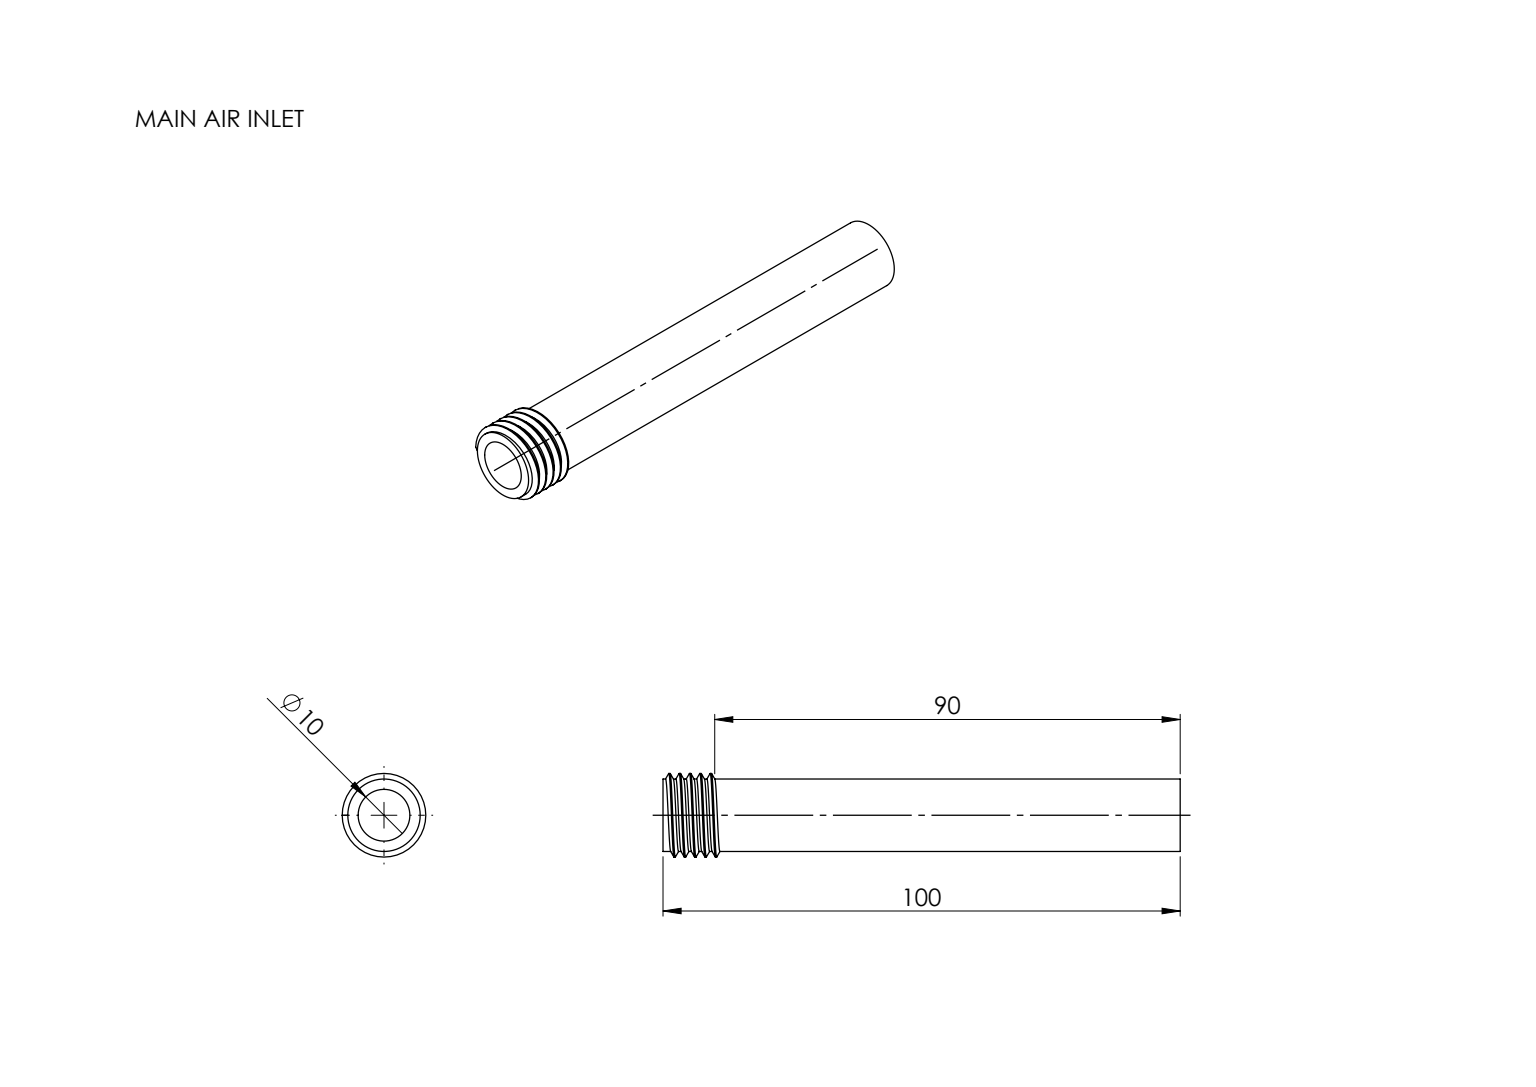
ISO-10303-21;
HEADER;
FILE_DESCRIPTION (('STEP AP214'),
    '1' );
FILE_NAME ('main air inlet.step',
    '2026-10-01T14:18:43',
    ( '' ),
    ( '' ),
    'SwSTEP 2.0',
    'SolidWorks 2026',
    '' );
FILE_SCHEMA (( 'AUTOMOTIVE_DESIGN' ));
ENDSEC;

DATA;
#5=CARTESIAN_POINT ( 'NONE',  ( 95.67376207875069838, 115.9545556584642867, -49.30000000000000426 ) ) ;
#31=CARTESIAN_POINT ( 'NONE',  ( 93.46109445667489979, 105.2492070361643215, -47.42499999726882720 ) ) ;
#33=CARTESIAN_POINT ( 'NONE',  ( 95.00472066334982912, 103.1245878333314323, -47.57499999726882578 ) ) ;
#51=CYLINDRICAL_SURFACE ( 'NONE', #259, 5.000000000000004441 ) ;
#69=CARTESIAN_POINT ( 'NONE',  ( 97.50236033167490746, 102.3130555110000159, -55.22499999726881725 ) ) ;
#81=CARTESIAN_POINT ( 'NONE',  ( 99.99999999999998579, 110.0000000000000000, -145.0000000000000284 ) ) ;
#106=ORIENTED_EDGE ( 'NONE', *, *, #13267, .T. ) ;
#118=EDGE_CURVE ( 'NONE', #27220, #19908, #1908, .T. ) ;
#123=CARTESIAN_POINT ( 'NONE',  ( 92.99999999999998579, 110.0000000000000000, -48.49999999453763877 ) ) ;
#146=CARTESIAN_POINT ( 'NONE',  ( 99.99999999999997158, 102.6397644303321215, -52.50000000000000711 ) ) ;
#174=CARTESIAN_POINT ( 'NONE',  ( 99.99999999999997158, 118.4984768113314146, -52.12499999726881583 ) ) ;
#176=CARTESIAN_POINT ( 'NONE',  ( 106.5389055433250860, 114.7507929638356785, -50.67499999726882010 ) ) ;
#194=CARTESIAN_POINT ( 'NONE',  ( 92.99999999999998579, 110.0000000000000000, -145.0000000000000284 ) ) ;
#209=CARTESIAN_POINT ( 'NONE',  ( 99.99999999999997158, 118.4984768113314004, -52.12499999726880873 ) ) ;
#217=ORIENTED_EDGE ( 'NONE', *, *, #21157, .F. ) ;
#223=CARTESIAN_POINT ( 'NONE',  ( 92.99999999999998579, 110.0000000000000000, -45.00000000000001421 ) ) ;
#257=CARTESIAN_POINT ( 'NONE',  ( 104.9952793366501567, 116.8754121666685393, -48.57499999726882578 ) ) ;
#259=AXIS2_PLACEMENT_3D ( 'NONE', #9021, #6875, #19848 ) ;
#265=CARTESIAN_POINT ( 'NONE',  ( 95.67376207875072680, 104.0454443415356991, -48.19999999453764161 ) ) ;
#289=CARTESIAN_POINT ( 'NONE',  ( 92.99999999999998579, 110.0000000000000000, -53.00000000000001421 ) ) ;
#301=CARTESIAN_POINT ( 'NONE',  ( 92.99999999999998579, 110.0000000000000000, -145.0000000000000284 ) ) ;
#315=CARTESIAN_POINT ( 'NONE',  ( 106.5389055433250860, 105.2492070361643215, -50.82499999726882578 ) ) ;
#317=CARTESIAN_POINT ( 'NONE',  ( 108.0825317499999869, 107.3738262389971538, -54.97499999726881015 ) ) ;
#353=CARTESIAN_POINT ( 'NONE',  ( 93.46109445667489979, 105.2492070361643215, -55.42499999726882720 ) ) ;
#376=ORIENTED_EDGE ( 'NONE', *, *, #19099, .T. ) ;
#388=LINE ( 'NONE', #2390, #9039 ) ;
#389=CARTESIAN_POINT ( 'NONE',  ( 95.67376207875072680, 115.9545556584642867, -54.79999999453764303 ) ) ;
#393=CARTESIAN_POINT ( 'NONE',  ( 106.9999999999999858, 112.2744378736303474, -51.90000000000001279 ) ) ;
#403=CARTESIAN_POINT ( 'NONE',  ( 102.4976396683250783, 117.6869444889999841, -46.47499999726882436 ) ) ;
#431=CARTESIAN_POINT ( 'NONE',  ( 95.67376207875069838, 115.9545556584642867, -47.30000000000000426 ) ) ;
#458=CARTESIAN_POINT ( 'NONE',  ( 97.50236033167490746, 117.6869444889999841, -50.02499999726882152 ) ) ;
#461=CARTESIAN_POINT ( 'NONE',  ( 92.99999999999998579, 110.0000000000000000, -48.49999999453763877 ) ) ;
#498=CARTESIAN_POINT ( 'NONE',  ( 91.91746824999998466, 110.0000000000000000, -53.62499999726882294 ) ) ;
#499=VERTEX_POINT ( 'NONE', #223 ) ;
#530=CARTESIAN_POINT ( 'NONE',  ( 107.0000000000000000, 110.0000000000000000, -55.49999999453763877 ) ) ;
#576=CARTESIAN_POINT ( 'NONE',  ( 95.67376207875069838, 104.0454443415356991, -50.70000000000000284 ) ) ;
#583=ORIENTED_EDGE ( 'NONE', *, *, #5538, .F. ) ;
#600=CARTESIAN_POINT ( 'NONE',  ( 95.00472066334981491, 103.1245878333314465, -51.32499999726881157 ) ) ;
#640=CARTESIAN_POINT ( 'NONE',  ( 102.4976396683250783, 117.6869444889999841, -50.47499999726882436 ) ) ;
#642=VECTOR ( 'NONE', #23365, 1000.000000000000000 ) ;
#674=CARTESIAN_POINT ( 'NONE',  ( 97.83688103937535629, 116.6573956140660897, -52.89999999453764445 ) ) ;
#679=CARTESIAN_POINT ( 'NONE',  ( 104.3262379212492448, 115.9545556584642867, -51.70000000000001705 ) ) ;
#688=CARTESIAN_POINT ( 'NONE',  ( 99.99999999999997158, 101.5015231886685712, -53.37499999726883004 ) ) ;
#699=CARTESIAN_POINT ( 'NONE',  ( 94.33688103937534208, 114.1144967660473242, -45.20000000000000995 ) ) ;
#714=CARTESIAN_POINT ( 'NONE',  ( 97.83688103937535629, 116.6573956140660897, -47.40000000000001279 ) ) ;
#718=CARTESIAN_POINT ( 'NONE',  ( 91.91746824999997045, 112.6261737610028320, -45.72499999726882436 ) ) ;
#722=ORIENTED_EDGE ( 'NONE', *, *, #13713, .T. ) ;
#785=CARTESIAN_POINT ( 'NONE',  ( 97.50236033167490746, 102.3130555110000159, -51.47499999726882436 ) ) ;
#789=VERTEX_POINT ( 'NONE', #17249 ) ;
#836=CARTESIAN_POINT ( 'NONE',  ( 108.0825317499999869, 107.3738262389971680, -54.97499999726881015 ) ) ;
#840=CARTESIAN_POINT ( 'NONE',  ( 99.99999999999997158, 102.6397644303321215, -52.50000000000000711 ) ) ;
#863=CARTESIAN_POINT ( 'NONE',  ( 92.99999999999998579, 110.0000000000000000, -54.49999999453763877 ) ) ;
#868=CARTESIAN_POINT ( 'NONE',  ( 97.50236033167490746, 117.6869444889999841, -50.02499999726882152 ) ) ;
#928=CARTESIAN_POINT ( 'NONE',  ( 93.46109445667489979, 114.7507929638356785, -48.07499999726882578 ) ) ;
#939=DIRECTION ( 'NONE',  ( 1.000000000000000000, 0.000000000000000000, 0.000000000000000000 ) ) ;
#956=EDGE_CURVE ( 'NONE', #3776, #27236, #5144, .T. ) ;
#960=CARTESIAN_POINT ( 'NONE',  ( 92.99999999999998579, 110.0000000000000000, -53.00000000000001421 ) ) ;
#979=CARTESIAN_POINT ( 'NONE',  ( 91.91746824999997045, 112.6261737610028320, -53.97499999726881725 ) ) ;
#1001=CARTESIAN_POINT ( 'NONE',  ( 93.00000000000000000, 112.2744378736303332, -46.59999999453763309 ) ) ;
#1011=CARTESIAN_POINT ( 'NONE',  ( 97.50236033167490746, 117.6869444889999841, -48.02499999726882152 ) ) ;
#1036=CARTESIAN_POINT ( 'NONE',  ( 108.0825317499999869, 112.6261737610028320, -54.52499999726881441 ) ) ;
#1059=DIRECTION ( 'NONE',  ( -1.000000000000000000, 0.000000000000000000, 0.000000000000000000 ) ) ;
#1071=CARTESIAN_POINT ( 'NONE',  ( 106.5389055433250860, 114.7507929638356785, -46.67499999726882720 ) ) ;
#1075=CARTESIAN_POINT ( 'NONE',  ( 107.0000000000000000, 112.2744378736303332, -45.89999999999999858 ) ) ;
#1118=CARTESIAN_POINT ( 'NONE',  ( 91.91746824999997045, 112.6261737610028320, -51.97499999726882436 ) ) ;
#1141=CARTESIAN_POINT ( 'NONE',  ( 107.0000000000000000, 110.0000000000000000, -46.00000000000001421 ) ) ;
#1144=CARTESIAN_POINT ( 'NONE',  ( 102.4976396683250783, 117.6869444889999841, -54.47499999726881725 ) ) ;
#1154=CARTESIAN_POINT ( 'NONE',  ( 104.3262379212492448, 115.9545556584642867, -53.70000000000000284 ) ) ;
#1213=CARTESIAN_POINT ( 'NONE',  ( 108.0825317500000011, 110.0000000000000000, -46.87499999726882294 ) ) ;
#1227=CIRCLE ( 'NONE', #17124, 7.000000000000006217 ) ;
#1256=CARTESIAN_POINT ( 'NONE',  ( 93.46109445667489979, 114.7507929638356785, -52.07499999726881867 ) ) ;
#1274=CARTESIAN_POINT ( 'NONE',  ( 104.3262379212492448, 104.0454443415356991, -46.30000000000001137 ) ) ;
#1277=CARTESIAN_POINT ( 'NONE',  ( 99.99999999999997158, 118.4984768113314004, -54.37499999726880873 ) ) ;
#1285=CARTESIAN_POINT ( 'NONE',  ( 102.4976396683250783, 102.3130555110000159, -47.02499999726882152 ) ) ;
#1289=ORIENTED_EDGE ( 'NONE', *, *, #10160, .T. ) ;
#1354=STYLED_ITEM ( 'NONE', ( #12417 ), #7649 ) ;
#1380=CARTESIAN_POINT ( 'NONE',  ( 97.50236033167490746, 117.6869444889999841, -46.02499999726882152 ) ) ;
#1418=CARTESIAN_POINT ( 'NONE',  ( 92.99999999999998579, 110.0000000000000000, -52.49999999453763877 ) ) ;
#1428=VERTEX_POINT ( 'NONE', #14617 ) ;
#1458=ORIENTED_EDGE ( 'NONE', *, *, #9332, .T. ) ;
#1473=CARTESIAN_POINT ( 'NONE',  ( 93.00000000000001421, 107.7255621263696241, -50.90000000000001279 ) ) ;
#1487=CARTESIAN_POINT ( 'NONE',  ( 102.4976396683250783, 102.3130555110000159, -53.27499999726882862 ) ) ;
#1492=EDGE_CURVE ( 'NONE', #8895, #21015, #19189, .T. ) ;
#1548=CARTESIAN_POINT ( 'NONE',  ( 104.3262379212492448, 104.0454443415356991, -49.79999999453762882 ) ) ;
#1559=CARTESIAN_POINT ( 'NONE',  ( 107.0000000000000000, 107.7255621263696668, -49.59999999453764019 ) ) ;
#1563=CARTESIAN_POINT ( 'NONE',  ( 93.00000000000001421, 107.7255621263696241, -52.39999999453765156 ) ) ;
#1568=CARTESIAN_POINT ( 'NONE',  ( 106.5389055433250860, 105.2492070361643215, -54.82499999726882578 ) ) ;
#1575=CARTESIAN_POINT ( 'NONE',  ( 92.99999999999998579, 110.0000000000000000, -145.0000000000000284 ) ) ;
#1600=ADVANCED_FACE ( 'NONE', ( #7157 ), #15853, .T. ) ;
#1651=CARTESIAN_POINT ( 'NONE',  ( 106.5389055433250860, 114.7507929638356785, -46.42499999726882720 ) ) ;
#1652=EDGE_LOOP ( 'NONE', ( #21390, #1458 ) ) ;
#1665=VECTOR ( 'NONE', #12127, 1000.000000000000000 ) ;
#1675=EDGE_CURVE ( 'NONE', #8859, #12248, #1227, .T. ) ;
#1689=DIRECTION ( 'NONE',  ( 5.782411586589358625E-17, -0.000000000000000000, 1.000000000000000000 ) ) ;
#1691=CIRCLE ( 'NONE', #24441, 7.000000000000006217 ) ;
#1694=CARTESIAN_POINT ( 'NONE',  ( 107.0000000000000000, 110.0000000000000000, -53.49999999453763877 ) ) ;
#1702=CARTESIAN_POINT ( 'NONE',  ( 106.5389055433250860, 114.7507929638356785, -50.42499999726882010 ) ) ;
#1710=EDGE_CURVE ( 'NONE', #11248, #1428, #16566, .T. ) ;
#1732=CARTESIAN_POINT ( 'NONE',  ( 107.0000000000000000, 107.7255621263696668, -46.10000000000000142 ) ) ;
#1749=DIRECTION ( 'NONE',  ( -0.000000000000000000, -0.000000000000000000, -1.000000000000000000 ) ) ;
#1764=CARTESIAN_POINT ( 'NONE',  ( 93.46109445667489979, 105.2492070361643215, -55.67499999726882720 ) ) ;
#1772=ORIENTED_EDGE ( 'NONE', *, *, #956, .T. ) ;
#1779=CARTESIAN_POINT ( 'NONE',  ( 104.3262379212492448, 115.9545556584642867, -47.19999999453763451 ) ) ;
#1829=EDGE_CURVE ( 'NONE', #20267, #3776, #7205, .T. ) ;
#1832=CARTESIAN_POINT ( 'NONE',  ( 95.67376207875069838, 115.9545556584642867, -54.79999999453764303 ) ) ;
#1842=CARTESIAN_POINT ( 'NONE',  ( 104.9952793366501709, 103.1245878333314323, -54.92499999726882720 ) ) ;
#1849=CARTESIAN_POINT ( 'NONE',  ( 107.0000000000000000, 110.0000000000000000, -52.00000000000001421 ) ) ;
#1873=CARTESIAN_POINT ( 'NONE',  ( 97.83688103937537051, 103.3426043859339103, -46.60000000000000853 ) ) ;
#1900=CARTESIAN_POINT ( 'NONE',  ( 91.91746824999997045, 107.3738262389971538, -47.77499999726880731 ) ) ;
#1908=( BOUNDED_CURVE ( )  B_SPLINE_CURVE ( 2, ( #9226, #22347, #21928, #19919, #17490, #13339, #403, #26188, #17781, #11486, #9086, #2404, #6798, #6519, #20202, #15340, #26629, #26484, #6654, #24055, #8661, #15484, #19774, #6939, #4677, #26049, #22066, #257, #4965, #8941, #7077, #15194, #10925, #23912, #13482, #4393, #21785, #17630, #2265, #15635, #2544, #11205, #24335, #4822, #7506, #18057, #9505, #26772, #12046, #9363, #7654, #5529, #24624, #27336, #14195, #7216, #20635, #22914, #11912, #12184, #18495, #1118, #1256, #25179, #5667, #3376, #20771, #20351, #9646, #15906, #20496, #3526, #5101, #18206, #18633, #688, #2954, #9917, #23051, #14056, #7796, #979, #13908, #7360, #16483, #14331, #5243, #9786, #26915, #5386, #27202, #836, #16346, #13765, #25045, #22636, #27056, #22488, #11627, #16053, #24763 ),
 .UNSPECIFIED., .F., .T. ) 
 B_SPLINE_CURVE_WITH_KNOTS ( ( 3, 2, 2, 2, 2, 2, 2, 2, 2, 2, 2, 2, 2, 2, 2, 2, 2, 2, 2, 2, 2, 2, 2, 2, 2, 2, 2, 2, 2, 2, 2, 2, 2, 2, 2, 2, 2, 2, 2, 2, 2, 2, 2, 2, 2, 2, 2, 2, 2, 2, 3 ),
 ( 0.000000000000000000, 0.02000000000000000042, 0.04000000000000000083, 0.05999999999999999778, 0.08000000000000000167, 0.1000000000000000056, 0.1199999999999999956, 0.1400000000000000133, 0.1600000000000000033, 0.1799999999999999933, 0.2000000000000000111, 0.2200000000000000011, 0.2399999999999999911, 0.2600000000000000089, 0.2800000000000000266, 0.2999999999999999889, 0.3200000000000000067, 0.3400000000000000244, 0.3599999999999999867, 0.3800000000000000044, 0.4000000000000000222, 0.4199999999999999845, 0.4400000000000000022, 0.4600000000000000200, 0.4799999999999999822, 0.5000000000000000000, 0.5200000000000000178, 0.5400000000000000355, 0.5600000000000000533, 0.5799999999999999600, 0.5999999999999999778, 0.6199999999999999956, 0.6400000000000000133, 0.6600000000000000311, 0.6800000000000000488, 0.6999999999999999556, 0.7199999999999999734, 0.7399999999999999911, 0.7600000000000000089, 0.7800000000000000266, 0.8000000000000000444, 0.8199999999999999512, 0.8399999999999999689, 0.8599999999999999867, 0.8800000000000000044, 0.9000000000000000222, 0.9200000000000000400, 0.9399999999999999467, 0.9599999999999999645, 0.9799999999999999822, 1.000000000000000000 ),
 .UNSPECIFIED. ) 
 CURVE ( )  GEOMETRIC_REPRESENTATION_ITEM ( )  RATIONAL_B_SPLINE_CURVE ( ( 1.000000000000000000, 0.9510565162951535312, 1.000000000000000000, 0.9510565162951535312, 1.000000000000000000, 0.9510565162951535312, 1.000000000000000000, 0.9510565162951535312, 1.000000000000000000, 0.9510565162951535312, 1.000000000000000000, 0.9510565162951535312, 1.000000000000000000, 0.9510565162951535312, 1.000000000000000000, 0.9510565162951535312, 1.000000000000000000, 0.9510565162951535312, 1.000000000000000000, 0.9510565162951535312, 1.000000000000000000, 0.9510565162951535312, 1.000000000000000000, 0.9510565162951535312, 1.000000000000000000, 0.9510565162951535312, 1.000000000000000000, 0.9510565162951535312, 1.000000000000000000, 0.9510565162951535312, 1.000000000000000000, 0.9510565162951535312, 1.000000000000000000, 0.9510565162951535312, 1.000000000000000000, 0.9510565162951535312, 1.000000000000000000, 0.9510565162951535312, 1.000000000000000000, 0.9510565162951535312, 1.000000000000000000, 0.9510565162951535312, 1.000000000000000000, 0.9510565162951535312, 1.000000000000000000, 0.9510565162951535312, 1.000000000000000000, 0.9510565162951535312, 1.000000000000000000, 0.9510565162951535312, 1.000000000000000000, 0.9510565162951535312, 1.000000000000000000, 0.9510565162951535312, 1.000000000000000000, 0.9510565162951535312, 1.000000000000000000, 0.9510565162951535312, 1.000000000000000000, 0.9510565162951535312, 1.000000000000000000, 0.9510565162951535312, 1.000000000000000000, 0.9510565162951535312, 1.000000000000000000, 0.9510565162951535312, 1.000000000000000000, 0.9510565162951535312, 1.000000000000000000, 0.9510565162951535312, 1.000000000000000000, 0.9510565162951535312, 1.000000000000000000, 0.9510565162951535312, 1.000000000000000000, 0.9510565162951535312, 1.000000000000000000, 0.9510565162951535312, 1.000000000000000000, 0.9510565162951535312, 1.000000000000000000, 0.9510565162951535312, 1.000000000000000000, 0.9510565162951535312, 1.000000000000000000, 0.9510565162951535312, 1.000000000000000000, 0.9510565162951535312, 1.000000000000000000, 0.9510565162951535312, 1.000000000000000000, 0.9510565162951535312, 1.000000000000000000, 0.9510565162951535312, 1.000000000000000000, 0.9510565162951535312, 1.000000000000000000, 0.9510565162951535312, 1.000000000000000000, 0.9510565162951535312, 1.000000000000000000 ) ) 
 REPRESENTATION_ITEM ( '' )  );
#1922=VERTEX_POINT ( 'NONE', #16975 ) ;
#1932=CARTESIAN_POINT ( 'NONE',  ( 91.91746824999997045, 112.6261737610028320, -47.72499999726881725 ) ) ;
#1964=FACE_OUTER_BOUND ( 'NONE', #11666, .T. ) ;
#1966=CARTESIAN_POINT ( 'NONE',  ( 97.83688103937537051, 103.3426043859339103, -54.09999999453764019 ) ) ;
#1969=CARTESIAN_POINT ( 'NONE',  ( 92.99999999999998579, 107.7255621263696526, -56.39999999453763024 ) ) ;
#1974=CARTESIAN_POINT ( 'NONE',  ( 102.4976396683250783, 117.6869444889999841, -50.22499999726882436 ) ) ;
#2032=ADVANCED_FACE ( 'NONE', ( #10693 ), #23546, .T. ) ;
#2033=CARTESIAN_POINT ( 'NONE',  ( 97.50236033167490746, 117.6869444889999841, -46.27499999726882152 ) ) ;
#2043=CARTESIAN_POINT ( 'NONE',  ( 92.99999999999998579, 107.7255621263696526, -54.90000000000001279 ) ) ;
#2067=CARTESIAN_POINT ( 'NONE',  ( 104.9952793366501709, 103.1245878333314323, -52.92499999726882010 ) ) ;
#2103=CARTESIAN_POINT ( 'NONE',  ( 92.99999999999998579, 110.0000000000000000, -56.49999999453763877 ) ) ;
#2118=DIRECTION ( 'NONE',  ( 5.782411586589358625E-17, -0.000000000000000000, 1.000000000000000000 ) ) ;
#2123=CARTESIAN_POINT ( 'NONE',  ( 94.33688103937535629, 105.8855032339526758, -48.29999999453764303 ) ) ;
#2147=CARTESIAN_POINT ( 'NONE',  ( 107.0000000000000000, 112.2744378736303332, -47.90000000000000568 ) ) ;
#2173=CARTESIAN_POINT ( 'NONE',  ( 104.9952793366501567, 103.1245878333314465, -48.92499999726882010 ) ) ;
#2175=CARTESIAN_POINT ( 'NONE',  ( 93.46109445667489979, 105.2492070361643215, -47.67499999726882720 ) ) ;
#2197=CARTESIAN_POINT ( 'NONE',  ( 99.99999999999998579, 110.0000000000000000, -145.0000000000000284 ) ) ;
#2201=ORIENTED_EDGE ( 'NONE', *, *, #6469, .F. ) ;
#2212=CARTESIAN_POINT ( 'NONE',  ( 102.4976396683250783, 102.3130555110000159, -55.02499999726882152 ) ) ;
#2265=CARTESIAN_POINT ( 'NONE',  ( 93.46109445667489979, 105.2492070361643215, -49.67499999726882010 ) ) ;
#2293=CARTESIAN_POINT ( 'NONE',  ( 107.0000000000000000, 107.7255621263696668, -52.10000000000001563 ) ) ;
#2318=CARTESIAN_POINT ( 'NONE',  ( 91.91746824999997045, 112.6261737610028320, -51.72499999726882436 ) ) ;
#2320=CARTESIAN_POINT ( 'NONE',  ( 91.91746824999998466, 110.0000000000000000, -47.87499999726882294 ) ) ;
#2355=CARTESIAN_POINT ( 'NONE',  ( 106.5389055433250860, 114.7507929638356785, -54.42499999726882720 ) ) ;
#2371=( BOUNDED_CURVE ( )  B_SPLINE_CURVE ( 2, ( #25636, #23648, #27790, #14928, #4123, #8248, #21506, #27653, #12788, #6119, #19361 ),
 .UNSPECIFIED., .F., .F. ) 
 B_SPLINE_CURVE_WITH_KNOTS ( ( 3, 2, 2, 2, 2, 3 ),
 ( 0.3000000000000002109, 0.3200000000000002287, 0.3400000000000003020, 0.3600000000000002642, 0.3800000000000003375, 0.4000000000000003553 ),
 .UNSPECIFIED. ) 
 CURVE ( )  GEOMETRIC_REPRESENTATION_ITEM ( )  RATIONAL_B_SPLINE_CURVE ( ( 0.9999999999999994449, 0.9510565162951540863, 1.000000000000000000, 0.9510565162951535312, 1.000000000000000000, 0.9510565162951535312, 1.000000000000000000, 0.9510565162951535312, 1.000000000000000000, 0.9510565162951527540, 1.000000000000000888 ) ) 
 REPRESENTATION_ITEM ( '' )  );
#2390=CARTESIAN_POINT ( 'NONE',  ( 107.0000000000000000, 110.0000000000000000, -145.0000000000000284 ) ) ;
#2394=ORIENTED_EDGE ( 'NONE', *, *, #2626, .F. ) ;
#2404=CARTESIAN_POINT ( 'NONE',  ( 108.0825317499999869, 107.3738262389971680, -46.97499999726881015 ) ) ;
#2433=CARTESIAN_POINT ( 'NONE',  ( 94.33688103937534208, 114.1144967660473242, -47.20000000000000995 ) ) ;
#2454=CARTESIAN_POINT ( 'NONE',  ( 97.50236033167490746, 102.3130555110000159, -49.22499999726882436 ) ) ;
#2456=CARTESIAN_POINT ( 'NONE',  ( 97.50236033167490746, 117.6869444889999841, -48.27499999726882152 ) ) ;
#2490=CARTESIAN_POINT ( 'NONE',  ( 91.91746824999997045, 112.6261737610028320, -51.72499999726882436 ) ) ;
#2544=CARTESIAN_POINT ( 'NONE',  ( 91.91746824999998466, 110.0000000000000000, -49.87499999726882294 ) ) ;
#2574=CARTESIAN_POINT ( 'NONE',  ( 99.99999999999997158, 117.3602355696678501, -51.50000000000001421 ) ) ;
#2581=VERTEX_POINT ( 'NONE', #10035 ) ;
#2599=CARTESIAN_POINT ( 'NONE',  ( 104.9952793366501567, 116.8754121666685393, -48.32499999726882578 ) ) ;
#2601=CARTESIAN_POINT ( 'NONE',  ( 95.67376207875069838, 104.0454443415356991, -48.19999999453764161 ) ) ;
#2626=EDGE_CURVE ( 'NONE', #499, #9571, #1691, .T. ) ;
#2635=CARTESIAN_POINT ( 'NONE',  ( 99.99999999999997158, 101.5015231886685854, -55.12499999726880873 ) ) ;
#2717=CARTESIAN_POINT ( 'NONE',  ( 107.0000000000000000, 107.7255621263696668, -50.10000000000001563 ) ) ;
#2738=CARTESIAN_POINT ( 'NONE',  ( 97.50236033167490746, 102.3130555110000159, -47.22499999726881725 ) ) ;
#2775=CARTESIAN_POINT ( 'NONE',  ( 99.99999999999997158, 118.4984768113314004, -50.37499999726881583 ) ) ;
#2822=CARTESIAN_POINT ( 'NONE',  ( 107.0000000000000000, 110.0000000000000000, -52.00000000000001421 ) ) ;
#2848=CARTESIAN_POINT ( 'NONE',  ( 99.99999999999997158, 102.6397644303321215, -54.50000000000000711 ) ) ;
#2909=CARTESIAN_POINT ( 'NONE',  ( 108.0825317499999869, 107.3738262389971538, -50.97499999726881015 ) ) ;
#2926=VERTEX_POINT ( 'NONE', #12931 ) ;
#2954=CARTESIAN_POINT ( 'NONE',  ( 97.50236033167490746, 102.3130555110000159, -53.47499999726882436 ) ) ;
#2971=EDGE_CURVE ( 'NONE', #1428, #24121, #25364, .T. ) ;
#2974=ORIENTED_EDGE ( 'NONE', *, *, #1675, .F. ) ;
#2986=CARTESIAN_POINT ( 'NONE',  ( 95.00472066334982912, 103.1245878333314323, -49.32499999726881157 ) ) ;
#2997=EDGE_LOOP ( 'NONE', ( #217, #7719, #21919, #9314 ) ) ;
#3015=CARTESIAN_POINT ( 'NONE',  ( 108.0825317500000011, 110.0000000000000000, -52.62499999726882294 ) ) ;
#3018=DIRECTION ( 'NONE',  ( -1.000000000000000000, 0.000000000000000000, 0.000000000000000000 ) ) ;
#3026=ORIENTED_EDGE ( 'NONE', *, *, #8370, .T. ) ;
#3054=CARTESIAN_POINT ( 'NONE',  ( 91.91746824999997045, 112.6261737610028320, -47.97499999726881725 ) ) ;
#3055=ADVANCED_FACE ( 'NONE', ( #23175 ), #17026, .F. ) ;
#3067=FACE_OUTER_BOUND ( 'NONE', #7175, .T. ) ;
#3079=ORIENTED_EDGE ( 'NONE', *, *, #10203, .T. ) ;
#3108=CARTESIAN_POINT ( 'NONE',  ( 97.83688103937537051, 103.3426043859339103, -52.60000000000001563 ) ) ;
#3130=CARTESIAN_POINT ( 'NONE',  ( 108.0825317500000011, 110.0000000000000000, -54.87499999726882294 ) ) ;
#3138=CARTESIAN_POINT ( 'NONE',  ( 95.00472066334982912, 103.1245878333314323, -47.32499999726881157 ) ) ;
#3161=CARTESIAN_POINT ( 'NONE',  ( 106.5389055433250860, 105.2492070361643215, -54.82499999726882578 ) ) ;
#3194=CARTESIAN_POINT ( 'NONE',  ( 104.9952793366501709, 116.8754121666685393, -52.57499999726881867 ) ) ;
#3253=CARTESIAN_POINT ( 'NONE',  ( 105.6631189606246153, 114.1144967660473242, -51.29999999453763593 ) ) ;
#3269=CARTESIAN_POINT ( 'NONE',  ( 91.91746824999998466, 110.0000000000000000, -53.87499999726882294 ) ) ;
#3277=CARTESIAN_POINT ( 'NONE',  ( 107.0000000000000000, 110.0000000000000000, -54.00000000000001421 ) ) ;
#3302=CARTESIAN_POINT ( 'NONE',  ( 91.91746824999998466, 110.0000000000000000, -53.62499999726882294 ) ) ;
#3307=AXIS2_PLACEMENT_3D ( 'NONE', #21369, #2118, #28196 ) ;
#3322=CARTESIAN_POINT ( 'NONE',  ( 104.3262379212492448, 104.0454443415356991, -50.30000000000001137 ) ) ;
#3335=CARTESIAN_POINT ( 'NONE',  ( 104.9952793366501709, 116.8754121666685393, -46.57499999726881157 ) ) ;
#3337=VERTEX_POINT ( 'NONE', #15403 ) ;
#3376=CARTESIAN_POINT ( 'NONE',  ( 99.99999999999997158, 118.4984768113314146, -52.37499999726881583 ) ) ;
#3377=ORIENTED_EDGE ( 'NONE', *, *, #20172, .T. ) ;
#3402=CARTESIAN_POINT ( 'NONE',  ( 102.4976396683250783, 102.3130555110000159, -53.27499999726882862 ) ) ;
#3404=EDGE_LOOP ( 'NONE', ( #14988, #8739, #722, #24690 ) ) ;
#3412=CARTESIAN_POINT ( 'NONE',  ( 106.5389055433250860, 114.7507929638356785, -46.42499999726882720 ) ) ;
#3430=DIRECTION ( 'NONE',  ( 5.782411586589358625E-17, -0.000000000000000000, 1.000000000000000000 ) ) ;
#3521=DIRECTION ( 'NONE',  ( 0.000000000000000000, 0.000000000000000000, -1.000000000000000000 ) ) ;
#3526=CARTESIAN_POINT ( 'NONE',  ( 108.0825317499999869, 107.3738262389971680, -52.97499999726881725 ) ) ;
#3550=CARTESIAN_POINT ( 'NONE',  ( 107.0000000000000000, 107.7255621263696668, -47.59999999453764019 ) ) ;
#3552=ORIENTED_EDGE ( 'NONE', *, *, #25847, .T. ) ;
#3558=CARTESIAN_POINT ( 'NONE',  ( 97.50236033167490746, 102.3130555110000159, -55.22499999726881725 ) ) ;
#3634=CARTESIAN_POINT ( 'NONE',  ( 107.0000000000000000, 110.0000000000000000, -47.49999999453763877 ) ) ;
#3649=CARTESIAN_POINT ( 'NONE',  ( 102.4976396683250783, 117.6869444889999841, -46.22499999726882436 ) ) ;
#3657=( BOUNDED_CURVE ( )  B_SPLINE_CURVE ( 2, ( #13324, #22189, #21916, #389, #4380, #21772, #10771, #17905, #9071, #26176, #530 ),
 .UNSPECIFIED., .F., .F. ) 
 B_SPLINE_CURVE_WITH_KNOTS ( ( 3, 2, 2, 2, 2, 3 ),
 ( 0.8000000000000000444, 0.8199999999999999512, 0.8399999999999999689, 0.8599999999999999867, 0.8800000000000000044, 0.9000000000000000222 ),
 .UNSPECIFIED. ) 
 CURVE ( )  GEOMETRIC_REPRESENTATION_ITEM ( )  RATIONAL_B_SPLINE_CURVE ( ( 1.000000000000000000, 0.9510565162951535312, 1.000000000000000000, 0.9510565162951535312, 1.000000000000000000, 0.9510565162951535312, 1.000000000000000000, 0.9510565162951535312, 1.000000000000000000, 0.9510565162951535312, 1.000000000000000000 ) ) 
 REPRESENTATION_ITEM ( '' )  );
#3678=CARTESIAN_POINT ( 'NONE',  ( 94.33688103937535629, 105.8855032339526758, -50.29999999453763593 ) ) ;
#3686=CARTESIAN_POINT ( 'NONE',  ( 95.67376207875072680, 104.0454443415356991, -46.70000000000000284 ) ) ;
#3688=DIRECTION ( 'NONE',  ( 5.782411586589358625E-17, -0.000000000000000000, 1.000000000000000000 ) ) ;
#3689=CARTESIAN_POINT ( 'NONE',  ( 94.33688103937534208, 114.1144967660473242, -52.69999999453764161 ) ) ;
#3699=CARTESIAN_POINT ( 'NONE',  ( 108.0825317499999869, 107.3738262389971538, -54.72499999726881015 ) ) ;
#3707=DIRECTION ( 'NONE',  ( 5.782411586589358625E-17, -0.000000000000000000, 1.000000000000000000 ) ) ;
#3729=EDGE_CURVE ( 'NONE', #23665, #499, #24540, .T. ) ;
#3733=ORIENTED_EDGE ( 'NONE', *, *, #2971, .F. ) ;
#3741=EDGE_LOOP ( 'NONE', ( #13883, #19434, #3079, #22446, #17485 ) ) ;
#3759=CARTESIAN_POINT ( 'NONE',  ( 104.9952793366501709, 103.1245878333314323, -53.17499999726882010 ) ) ;
#3776=VERTEX_POINT ( 'NONE', #6135 ) ;
#3786=CARTESIAN_POINT ( 'NONE',  ( 91.91746824999997045, 112.6261737610028320, -49.72499999726881725 ) ) ;
#3795=CARTESIAN_POINT ( 'NONE',  ( 91.91746824999998466, 110.0000000000000000, -45.74999999726882294 ) ) ;
#3806=VECTOR ( 'NONE', #3707, 1000.000000000000000 ) ;
#3822=CARTESIAN_POINT ( 'NONE',  ( 107.0000000000000000, 112.2744378736303332, -49.39999999453763735 ) ) ;
#3830=CARTESIAN_POINT ( 'NONE',  ( 106.5389055433250860, 105.2492070361643215, -52.82499999726881867 ) ) ;
#3898=CYLINDRICAL_SURFACE ( 'NONE', #24842, 7.000000000000006217 ) ;
#3921=DIRECTION ( 'NONE',  ( -1.000000000000000000, 0.000000000000000000, 0.000000000000000000 ) ) ;
#3928=ADVANCED_FACE ( 'NONE', ( #16156 ), #9046, .T. ) ;
#3953=CARTESIAN_POINT ( 'NONE',  ( 93.00000000000001421, 107.7255621263696241, -50.39999999453763024 ) ) ;
#3963=AXIS2_PLACEMENT_3D ( 'NONE', #20723, #23383, #6408 ) ;
#3966=CARTESIAN_POINT ( 'NONE',  ( 93.00000000000000000, 112.2744378736303332, -50.59999999453763309 ) ) ;
#3974=CARTESIAN_POINT ( 'NONE',  ( 108.0825317500000011, 110.0000000000000000, -52.62499999726882294 ) ) ;
#4004=CARTESIAN_POINT ( 'NONE',  ( 104.3262379212492448, 104.0454443415356991, -46.30000000000001847 ) ) ;
#4007=DIRECTION ( 'NONE',  ( 5.782411586589358625E-17, -0.000000000000000000, 1.000000000000000000 ) ) ;
#4031=CARTESIAN_POINT ( 'NONE',  ( 104.9952793366501709, 103.1245878333314323, -47.17499999726881299 ) ) ;
#4033=( BOUNDED_CURVE ( )  B_SPLINE_CURVE ( 2, ( #1141, #7816, #5407, #1274, #20793, #18512, #14218, #3686, #14494, #27219, #11792 ),
 .UNSPECIFIED., .F., .F. ) 
 B_SPLINE_CURVE_WITH_KNOTS ( ( 3, 2, 2, 2, 2, 3 ),
 ( 0.1000000000000000056, 0.1200000000000000233, 0.1400000000000000688, 0.1600000000000001144, 0.1800000000000001044, 0.2000000000000001776 ),
 .UNSPECIFIED. ) 
 CURVE ( )  GEOMETRIC_REPRESENTATION_ITEM ( )  RATIONAL_B_SPLINE_CURVE ( ( 1.000000000000000000, 0.9510565162951535312, 1.000000000000000000, 0.9510565162951535312, 1.000000000000000000, 0.9510565162951535312, 1.000000000000000000, 0.9510565162951535312, 1.000000000000000000, 0.9510565162951530871, 1.000000000000000444 ) ) 
 REPRESENTATION_ITEM ( '' )  );
#4037=CARTESIAN_POINT ( 'NONE',  ( 106.5389055433250860, 105.2492070361643215, -53.07499999726881867 ) ) ;
#4066=MECHANICAL_DESIGN_GEOMETRIC_PRESENTATION_REPRESENTATION('',(#1354),#14062);
#4095=DIRECTION ( 'NONE',  ( 5.782411586589358625E-17, -0.000000000000000000, 1.000000000000000000 ) ) ;
#4102=CARTESIAN_POINT ( 'NONE',  ( 93.00000000000000000, 107.7255621263696526, -50.39999999453763024 ) ) ;
#4111=CARTESIAN_POINT ( 'NONE',  ( 97.50236033167490746, 102.3130555110000159, -53.22499999726882436 ) ) ;
#4118=ADVANCED_FACE ( 'NONE', ( #23667 ), #25775, .F. ) ;
#4123=CARTESIAN_POINT ( 'NONE',  ( 102.1631189606246295, 103.3426043859339103, -48.40000000000001279 ) ) ;
#4171=CARTESIAN_POINT ( 'NONE',  ( 95.00472066334982912, 116.8754121666685393, -46.17499999726882720 ) ) ;
#4179=CARTESIAN_POINT ( 'NONE',  ( 105.6631189606246295, 105.8855032339526758, -54.20000000000000995 ) ) ;
#4219=DIRECTION ( 'NONE',  ( -1.000000000000000000, 0.000000000000000000, 5.782411586589357392E-17 ) ) ;
#4226=CARTESIAN_POINT ( 'NONE',  ( 92.99999999999998579, 110.0000000000000000, -50.49999999453763877 ) ) ;
#4256=CARTESIAN_POINT ( 'NONE',  ( 102.1631189606246295, 103.3426043859339103, -47.89999999453763735 ) ) ;
#4280=CARTESIAN_POINT ( 'NONE',  ( 97.83688103937535629, 116.6573956140660897, -49.40000000000001279 ) ) ;
#4311=CARTESIAN_POINT ( 'NONE',  ( 102.4976396683250783, 102.3130555110000159, -49.27499999726882152 ) ) ;
#4327=DIRECTION ( 'NONE',  ( 1.000000000000000000, 0.000000000000000000, 0.000000000000000000 ) ) ;
#4333=SURFACE_SIDE_STYLE ('',( #23719 ) ) ;
#4340=VECTOR ( 'NONE', #20910, 1000.000000000000114 ) ;
#4343=CARTESIAN_POINT ( 'NONE',  ( 104.9952793366501709, 103.1245878333314323, -50.92499999726882010 ) ) ;
#4358=( BOUNDED_CURVE ( )  B_SPLINE_CURVE ( 2, ( #27634, #10080, #23217, #27771, #18792, #21355, #12356, #25208, #8093, #1563, #27225 ),
 .UNSPECIFIED., .F., .F. ) 
 B_SPLINE_CURVE_WITH_KNOTS ( ( 3, 2, 2, 2, 2, 3 ),
 ( 0.4999999999999996669, 0.5199999999999996847, 0.5399999999999998135, 0.5599999999999998312, 0.5799999999999998490, 0.5999999999999998668 ),
 .UNSPECIFIED. ) 
 CURVE ( )  GEOMETRIC_REPRESENTATION_ITEM ( )  RATIONAL_B_SPLINE_CURVE ( ( 1.000000000000000888, 0.9510565162951527540, 1.000000000000000000, 0.9510565162951535312, 1.000000000000000000, 0.9510565162951535312, 1.000000000000000000, 0.9510565162951535312, 1.000000000000000000, 0.9510565162951537532, 0.9999999999999997780 ) ) 
 REPRESENTATION_ITEM ( '' )  );
#4380=CARTESIAN_POINT ( 'NONE',  ( 97.83688103937535629, 116.6573956140660897, -54.89999999453763735 ) ) ;
#4393=CARTESIAN_POINT ( 'NONE',  ( 99.99999999999997158, 101.5015231886685712, -49.37499999726882294 ) ) ;
#4424=CARTESIAN_POINT ( 'NONE',  ( 104.3262379212492448, 115.9545556584642867, -51.70000000000001705 ) ) ;
#4449=CARTESIAN_POINT ( 'NONE',  ( 106.5389055433250860, 114.7507929638356785, -48.42499999726882010 ) ) ;
#4451=CARTESIAN_POINT ( 'NONE',  ( 104.9952793366501709, 116.8754121666685393, -48.57499999726881867 ) ) ;
#4486=CARTESIAN_POINT ( 'NONE',  ( 91.91746824999997045, 112.6261737610028320, -53.72499999726881725 ) ) ;
#4519=CARTESIAN_POINT ( 'NONE',  ( 104.3262379212492448, 115.9545556584642867, -49.70000000000001705 ) ) ;
#4539=CARTESIAN_POINT ( 'NONE',  ( 92.99999999999998579, 107.7255621263696952, -48.39999999453764445 ) ) ;
#4560=CARTESIAN_POINT ( 'NONE',  ( 94.33688103937534208, 114.1144967660473242, -49.20000000000001705 ) ) ;
#4576=AXIS2_PLACEMENT_3D ( 'NONE', #14901, #19337, #25611 ) ;
#4586=CARTESIAN_POINT ( 'NONE',  ( 102.4976396683250783, 117.6869444889999841, -52.22499999726882436 ) ) ;
#4588=CARTESIAN_POINT ( 'NONE',  ( 106.5389055433250860, 105.2492070361643215, -47.07499999726882578 ) ) ;
#4590=EDGE_CURVE ( 'NONE', #1922, #27220, #27600, .T. ) ;
#4607=ADVANCED_BREP_SHAPE_REPRESENTATION ( '', ( #7649, #26844 ), #10431 ) ;
#4626=CARTESIAN_POINT ( 'NONE',  ( 95.00472066334982912, 116.8754121666685393, -51.92499999726881299 ) ) ;
#4650=ORIENTED_EDGE ( 'NONE', *, *, #15930, .T. ) ;
#4662=CARTESIAN_POINT ( 'NONE',  ( 102.1631189606246295, 103.3426043859339103, -55.89999999453763735 ) ) ;
#4677=CARTESIAN_POINT ( 'NONE',  ( 97.50236033167490746, 117.6869444889999841, -48.27499999726882152 ) ) ;
#4707=CARTESIAN_POINT ( 'NONE',  ( 102.1631189606246295, 103.3426043859339103, -52.40000000000001279 ) ) ;
#4732=CARTESIAN_POINT ( 'NONE',  ( 93.46109445667489979, 114.7507929638356785, -49.82499999726882578 ) ) ;
#4734=CARTESIAN_POINT ( 'NONE',  ( 102.4976396683250783, 117.6869444889999841, -52.47499999726882436 ) ) ;
#4767=CARTESIAN_POINT ( 'NONE',  ( 97.50236033167490746, 102.3130555110000159, -51.22499999726882436 ) ) ;
#4809=CARTESIAN_POINT ( 'NONE',  ( 105.6631189606246153, 114.1144967660473242, -51.80000000000001137 ) ) ;
#4822=CARTESIAN_POINT ( 'NONE',  ( 95.00472066334981491, 116.8754121666685393, -50.17499999726882010 ) ) ;
#4852=CARTESIAN_POINT ( 'NONE',  ( 107.0000000000000000, 110.0000000000000000, -48.00000000000001421 ) ) ;
#4878=CARTESIAN_POINT ( 'NONE',  ( 106.5389055433250860, 114.7507929638356785, -50.42499999726882010 ) ) ;
#4880=CARTESIAN_POINT ( 'NONE',  ( 95.00472066334982912, 103.1245878333314323, -55.57499999726881157 ) ) ;
#4916=CARTESIAN_POINT ( 'NONE',  ( 106.5389055433250860, 105.2492070361643215, -50.82499999726882578 ) ) ;
#4965=CARTESIAN_POINT ( 'NONE',  ( 106.5389055433250860, 114.7507929638356785, -48.67499999726882010 ) ) ;
#4998=CARTESIAN_POINT ( 'NONE',  ( 93.00000000000000000, 107.7255621263696526, -54.90000000000001279 ) ) ;
#5020=CARTESIAN_POINT ( 'NONE',  ( 102.4976396683250783, 102.3130555110000159, -47.02499999726882152 ) ) ;
#5022=AXIS2_PLACEMENT_3D ( 'NONE', #13815, #3430, #9272 ) ;
#5055=CARTESIAN_POINT ( 'NONE',  ( 102.4976396683250783, 117.6869444889999841, -48.47499999726882436 ) ) ;
#5071=( BOUNDED_CURVE ( )  B_SPLINE_CURVE ( 2, ( #11165, #18133, #9434, #12532, #6147, #14676, #27542, #6012, #12258, #5602, #20848 ),
 .UNSPECIFIED., .F., .F. ) 
 B_SPLINE_CURVE_WITH_KNOTS ( ( 3, 2, 2, 2, 2, 3 ),
 ( 0.8000000000000000444, 0.8199999999999999512, 0.8399999999999999689, 0.8599999999999999867, 0.8800000000000000044, 0.9000000000000000222 ),
 .UNSPECIFIED. ) 
 CURVE ( )  GEOMETRIC_REPRESENTATION_ITEM ( )  RATIONAL_B_SPLINE_CURVE ( ( 1.000000000000000000, 0.9510565162951535312, 1.000000000000000000, 0.9510565162951535312, 1.000000000000000000, 0.9510565162951535312, 1.000000000000000000, 0.9510565162951535312, 1.000000000000000000, 0.9510565162951535312, 1.000000000000000000 ) ) 
 REPRESENTATION_ITEM ( '' )  );
#5101=CARTESIAN_POINT ( 'NONE',  ( 106.5389055433250860, 105.2492070361643215, -53.07499999726881867 ) ) ;
#5131=CARTESIAN_POINT ( 'NONE',  ( 95.00472066334982912, 116.8754121666685393, -47.92499999726882010 ) ) ;
#5144=LINE ( 'NONE', #301, #14401 ) ;
#5153=FACE_OUTER_BOUND ( 'NONE', #3404, .T. ) ;
#5159=CARTESIAN_POINT ( 'NONE',  ( 93.46109445667489979, 114.7507929638356785, -53.82499999726881867 ) ) ;
#5196=CARTESIAN_POINT ( 'NONE',  ( 95.00472066334982912, 116.8754121666685393, -50.17499999726882010 ) ) ;
#5200=ORIENTED_EDGE ( 'NONE', *, *, #16341, .F. ) ;
#5215=ORIENTED_EDGE ( 'NONE', *, *, #1492, .T. ) ;
#5224=CARTESIAN_POINT ( 'NONE',  ( 107.0000000000000000, 110.0000000000000000, -47.49999999453763877 ) ) ;
#5243=CARTESIAN_POINT ( 'NONE',  ( 102.4976396683250783, 117.6869444889999841, -54.47499999726881725 ) ) ;
#5268=CARTESIAN_POINT ( 'NONE',  ( 99.99999999999998579, 110.0000000000000000, -145.0000000000000284 ) ) ;
#5270=CARTESIAN_POINT ( 'NONE',  ( 105.6631189606246153, 114.1144967660473242, -47.80000000000001137 ) ) ;
#5274=CARTESIAN_POINT ( 'NONE',  ( 102.4976396683250783, 117.6869444889999841, -46.22499999726882436 ) ) ;
#5302=CARTESIAN_POINT ( 'NONE',  ( 102.4976396683250783, 102.3130555110000159, -53.02499999726882862 ) ) ;
#5339=CARTESIAN_POINT ( 'NONE',  ( 108.0825317499999869, 107.3738262389971538, -46.97499999726881015 ) ) ;
#5358=ORIENTED_EDGE ( 'NONE', *, *, #16341, .T. ) ;
#5386=CARTESIAN_POINT ( 'NONE',  ( 108.0825317499999869, 112.6261737610028320, -54.77499999726881441 ) ) ;
#5396=DIRECTION ( 'NONE',  ( 5.782411586589358625E-17, -0.000000000000000000, 1.000000000000000000 ) ) ;
#5407=CARTESIAN_POINT ( 'NONE',  ( 105.6631189606246295, 105.8855032339526758, -46.20000000000000995 ) ) ;
#5412=CARTESIAN_POINT ( 'NONE',  ( 93.46109445667489979, 105.2492070361643215, -53.67499999726882720 ) ) ;
#5421=CARTESIAN_POINT ( 'NONE',  ( 97.50236033167490746, 102.3130555110000159, -47.22499999726881725 ) ) ;
#5444=AXIS2_PLACEMENT_3D ( 'NONE', #8711, #21840, #21976 ) ;
#5458=STYLED_ITEM ( 'NONE', ( #10864 ), #4607 ) ;
#5478=CARTESIAN_POINT ( 'NONE',  ( 106.5389055433250860, 114.7507929638356785, -48.67499999726882010 ) ) ;
#5495=EDGE_CURVE ( 'NONE', #27220, #23665, #9503, .T. ) ;
#5501=ORIENTED_EDGE ( 'NONE', *, *, #12587, .T. ) ;
#5512=CARTESIAN_POINT ( 'NONE',  ( 106.9999999999999858, 112.2744378736303474, -53.39999999453764445 ) ) ;
#5529=CARTESIAN_POINT ( 'NONE',  ( 108.0825317499999869, 107.3738262389971680, -50.97499999726881725 ) ) ;
#5536=CARTESIAN_POINT ( 'NONE',  ( 94.33688103937534208, 114.1144967660473242, -50.69999999453764161 ) ) ;
#5538=EDGE_CURVE ( 'NONE', #2926, #21015, #20880, .T. ) ;
#5556=CARTESIAN_POINT ( 'NONE',  ( 106.5389055433250860, 105.2492070361643215, -55.07499999726882578 ) ) ;
#5565=CARTESIAN_POINT ( 'NONE',  ( 99.99999999999997158, 118.4984768113314004, -46.12499999726880873 ) ) ;
#5568=ORIENTED_EDGE ( 'NONE', *, *, #14474, .T. ) ;
#5588=CARTESIAN_POINT ( 'NONE',  ( 104.9952793366501567, 103.1245878333314465, -54.92499999726882720 ) ) ;
#5602=CARTESIAN_POINT ( 'NONE',  ( 107.0000000000000000, 112.2744378736303190, -53.90000000000000568 ) ) ;
#5608=CARTESIAN_POINT ( 'NONE',  ( 105.6631189606246295, 105.8855032339526758, -50.20000000000001705 ) ) ;
#5629=AXIS2_PLACEMENT_3D ( 'NONE', #9750, #16014, #939 ) ;
#5667=CARTESIAN_POINT ( 'NONE',  ( 97.50236033167490746, 117.6869444889999841, -52.27499999726882862 ) ) ;
#5674=DIRECTION ( 'NONE',  ( -0.000000000000000000, -0.000000000000000000, 1.000000000000000000 ) ) ;
#5691=CARTESIAN_POINT ( 'NONE',  ( 102.1631189606246295, 103.3426043859339103, -47.89999999453763735 ) ) ;
#5701=CARTESIAN_POINT ( 'NONE',  ( 91.91746824999998466, 110.0000000000000000, -53.62499999726882294 ) ) ;
#5756=SURFACE_STYLE_FILL_AREA ( #8433 ) ;
#5767=ORIENTED_EDGE ( 'NONE', *, *, #1710, .T. ) ;
#5790=CARTESIAN_POINT ( 'NONE',  ( 99.99999999999997158, 101.5015231886685854, -49.12499999726882294 ) ) ;
#5829=CARTESIAN_POINT ( 'NONE',  ( 95.67376207875069838, 115.9545556584642867, -50.79999999453764303 ) ) ;
#5837=CARTESIAN_POINT ( 'NONE',  ( 93.46109445667489979, 105.2492070361643215, -53.42499999726882720 ) ) ;
#5897=SURFACE_SIDE_STYLE ('',( #5756 ) ) ;
#5916=CARTESIAN_POINT ( 'NONE',  ( 95.67376207875072680, 115.9545556584642867, -46.79999999453764303 ) ) ;
#5928=CARTESIAN_POINT ( 'NONE',  ( 91.91746824999997045, 107.3738262389971538, -49.52499999726881441 ) ) ;
#5962=CARTESIAN_POINT ( 'NONE',  ( 97.83688103937537051, 103.3426043859339103, -52.09999999453764019 ) ) ;
#5972=CARTESIAN_POINT ( 'NONE',  ( 95.00472066334982912, 116.8754121666685393, -53.92499999726881299 ) ) ;
#6012=CARTESIAN_POINT ( 'NONE',  ( 104.3262379212492448, 115.9545556584642867, -53.69999999999999574 ) ) ;
#6040=CARTESIAN_POINT ( 'NONE',  ( 97.83688103937537051, 103.3426043859339103, -54.60000000000000853 ) ) ;
#6056=SURFACE_STYLE_USAGE ( .BOTH. , #4333 ) ;
#6064=CARTESIAN_POINT ( 'NONE',  ( 108.0825317499999869, 112.6261737610028320, -46.52499999726882152 ) ) ;
#6071=EDGE_CURVE ( 'NONE', #16704, #17997, #2371, .T. ) ;
#6079=DIRECTION ( 'NONE',  ( -5.782411586589357392E-17, 0.000000000000000000, -1.000000000000000000 ) ) ;
#6095=CYLINDRICAL_SURFACE ( 'NONE', #4576, 7.000000000000006217 ) ;
#6099=CARTESIAN_POINT ( 'NONE',  ( 107.0000000000000000, 110.0000000000000000, -49.49999999453764588 ) ) ;
#6107=CARTESIAN_POINT ( 'NONE',  ( 95.00472066334982912, 103.1245878333314323, -53.32499999726881157 ) ) ;
#6119=CARTESIAN_POINT ( 'NONE',  ( 92.99999999999997158, 107.7255621263696810, -48.90000000000001279 ) ) ;
#6135=CARTESIAN_POINT ( 'NONE',  ( 92.99999999999998579, 110.0000000000000000, -51.00000000000000711 ) ) ;
#6147=CARTESIAN_POINT ( 'NONE',  ( 97.83688103937535629, 116.6573956140660897, -53.40000000000001990 ) ) ;
#6164=CARTESIAN_POINT ( 'NONE',  ( 108.0825317499999869, 112.6261737610028320, -48.77499999726882152 ) ) ;
#6170=CARTESIAN_POINT ( 'NONE',  ( 91.91746824999997045, 107.3738262389971538, -55.77499999726882862 ) ) ;
#6200=CARTESIAN_POINT ( 'NONE',  ( 91.91746824999997045, 107.3738262389971538, -47.52499999726881441 ) ) ;
#6201=EDGE_CURVE ( 'NONE', #499, #21009, #7037, .T. ) ;
#6237=CARTESIAN_POINT ( 'NONE',  ( 99.99999999999997158, 117.3602355696678501, -54.99999999453763166 ) ) ;
#6241=CARTESIAN_POINT ( 'NONE',  ( 107.0000000000000000, 107.7255621263696668, -55.59999999453764019 ) ) ;
#6245=CARTESIAN_POINT ( 'NONE',  ( 91.91746824999997045, 112.6261737610028320, -51.72499999726882436 ) ) ;
#6298=CARTESIAN_POINT ( 'NONE',  ( 102.4976396683250783, 117.6869444889999841, -50.47499999726882436 ) ) ;
#6309=CARTESIAN_POINT ( 'NONE',  ( 92.99999999999998579, 110.0000000000000000, -55.00000000000002132 ) ) ;
#6333=CARTESIAN_POINT ( 'NONE',  ( 104.9952793366501709, 116.8754121666685393, -48.32499999726881867 ) ) ;
#6352=AXIS2_PLACEMENT_3D ( 'NONE', #20558, #16117, #3018 ) ;
#6371=CARTESIAN_POINT ( 'NONE',  ( 102.1631189606246295, 103.3426043859339103, -53.89999999453763735 ) ) ;
#6408=DIRECTION ( 'NONE',  ( -1.000000000000000000, 0.000000000000000000, 0.000000000000000000 ) ) ;
#6413=CARTESIAN_POINT ( 'NONE',  ( 95.67376207875069838, 115.9545556584642867, -51.30000000000000426 ) ) ;
#6433=( BOUNDED_CURVE ( )  B_SPLINE_CURVE ( 2, ( #9368, #9652, #5536, #25052, #22783, #18502, #7935, #18773, #3253, #7366, #7660 ),
 .UNSPECIFIED., .F., .F. ) 
 B_SPLINE_CURVE_WITH_KNOTS ( ( 3, 2, 2, 2, 2, 3 ),
 ( 0.3999999999999996891, 0.4199999999999996514, 0.4399999999999996692, 0.4599999999999996869, 0.4799999999999996492, 0.4999999999999996669 ),
 .UNSPECIFIED. ) 
 CURVE ( )  GEOMETRIC_REPRESENTATION_ITEM ( )  RATIONAL_B_SPLINE_CURVE ( ( 1.000000000000000888, 0.9510565162951527540, 1.000000000000000000, 0.9510565162951535312, 1.000000000000000000, 0.9510565162951535312, 1.000000000000000000, 0.9510565162951535312, 1.000000000000000000, 0.9510565162951543083, 0.9999999999999992228 ) ) 
 REPRESENTATION_ITEM ( '' )  );
#6440=CARTESIAN_POINT ( 'NONE',  ( 102.4976396683250783, 117.6869444889999841, -46.47499999726882436 ) ) ;
#6448=DIRECTION ( 'NONE',  ( 1.000000000000000000, 0.000000000000000000, 0.000000000000000000 ) ) ;
#6469=EDGE_CURVE ( 'NONE', #10849, #27236, #12847, .T. ) ;
#6472=CARTESIAN_POINT ( 'NONE',  ( 97.50236033167490746, 117.6869444889999841, -50.02499999726882152 ) ) ;
#6503=ORIENTED_EDGE ( 'NONE', *, *, #22032, .T. ) ;
#6519=CARTESIAN_POINT ( 'NONE',  ( 104.9952793366501567, 103.1245878333314465, -47.17499999726882010 ) ) ;
#6546=CARTESIAN_POINT ( 'NONE',  ( 93.00000000000000000, 112.2744378736303332, -51.10000000000000142 ) ) ;
#6570=CARTESIAN_POINT ( 'NONE',  ( 108.0825317499999869, 107.3738262389971680, -50.72499999726881725 ) ) ;
#6572=CARTESIAN_POINT ( 'NONE',  ( 91.91746824999997045, 107.3738262389971538, -49.77499999726881441 ) ) ;
#6581=PLANE ( 'NONE',  #10250 ) ;
#6607=CARTESIAN_POINT ( 'NONE',  ( 97.50236033167490746, 117.6869444889999841, -46.27499999726882152 ) ) ;
#6625=FACE_BOUND ( 'NONE', #1652, .T. ) ;
#6636=CARTESIAN_POINT ( 'NONE',  ( 92.99999999999998579, 110.0000000000000000, -145.0000000000000284 ) ) ;
#6654=CARTESIAN_POINT ( 'NONE',  ( 93.46109445667489979, 105.2492070361643215, -47.67499999726882720 ) ) ;
#6672=FACE_OUTER_BOUND ( 'NONE', #20087, .T. ) ;
#6677=ORIENTED_EDGE ( 'NONE', *, *, #5495, .F. ) ;
#6683=CARTESIAN_POINT ( 'NONE',  ( 107.0000000000000000, 110.0000000000000000, -52.00000000000001421 ) ) ;
#6697=EDGE_CURVE ( 'NONE', #499, #1922, #22610, .T. ) ;
#6710=CARTESIAN_POINT ( 'NONE',  ( 91.91746824999997045, 107.3738262389971680, -47.52499999726881441 ) ) ;
#6713=CARTESIAN_POINT ( 'NONE',  ( 99.99999999999997158, 101.5015231886685854, -51.37499999726882294 ) ) ;
#6749=CARTESIAN_POINT ( 'NONE',  ( 93.46109445667489979, 114.7507929638356785, -49.82499999726882578 ) ) ;
#6752=ORIENTED_EDGE ( 'NONE', *, *, #8600, .F. ) ;
#6798=CARTESIAN_POINT ( 'NONE',  ( 106.5389055433250860, 105.2492070361643215, -47.07499999726882578 ) ) ;
#6828=CARTESIAN_POINT ( 'NONE',  ( 97.83688103937535629, 116.6573956140660897, -47.40000000000001279 ) ) ;
#6833=ORIENTED_EDGE ( 'NONE', *, *, #13516, .T. ) ;
#6852=CARTESIAN_POINT ( 'NONE',  ( 91.91746824999998466, 110.0000000000000000, -47.62499999726882294 ) ) ;
#6854=CARTESIAN_POINT ( 'NONE',  ( 108.0825317499999869, 112.6261737610028320, -52.77499999726883573 ) ) ;
#6866=CARTESIAN_POINT ( 'NONE',  ( 94.33688103937534208, 114.1144967660473242, -48.69999999453764161 ) ) ;
#6875=DIRECTION ( 'NONE',  ( 5.782411586589358625E-17, -0.000000000000000000, 1.000000000000000000 ) ) ;
#6893=CARTESIAN_POINT ( 'NONE',  ( 106.5389055433250860, 114.7507929638356785, -50.42499999726882010 ) ) ;
#6924=CARTESIAN_POINT ( 'NONE',  ( 104.3262379212492448, 104.0454443415356991, -55.79999999453763593 ) ) ;
#6927=EDGE_CURVE ( 'NONE', #3337, #11248, #19368, .T. ) ;
#6939=CARTESIAN_POINT ( 'NONE',  ( 95.00472066334981491, 116.8754121666685393, -48.17499999726882010 ) ) ;
#6970=CARTESIAN_POINT ( 'NONE',  ( 94.33688103937535629, 105.8855032339526758, -46.80000000000001847 ) ) ;
#6994=CARTESIAN_POINT ( 'NONE',  ( 108.0825317499999869, 112.6261737610028320, -46.52499999726882152 ) ) ;
#6996=CARTESIAN_POINT ( 'NONE',  ( 95.67376207875069838, 115.9545556584642867, -46.79999999453764303 ) ) ;
#7003=CARTESIAN_POINT ( 'NONE',  ( 99.99999999999997158, 117.3602355696678643, -48.99999999453763877 ) ) ;
#7026=CARTESIAN_POINT ( 'NONE',  ( 91.91746824999998466, 110.0000000000000000, -45.87499999726882294 ) ) ;
#7031=ORIENTED_EDGE ( 'NONE', *, *, #9332, .F. ) ;
#7037=( BOUNDED_CURVE ( )  B_SPLINE_CURVE ( 2, ( #15496, #24489, #699, #22076, #7228, #19929, #15919, #9096, #19785, #13494, #17791 ),
 .UNSPECIFIED., .F., .T. ) 
 B_SPLINE_CURVE_WITH_KNOTS ( ( 3, 2, 2, 2, 2, 3 ),
 ( 0.000000000000000000, 0.02000000000000000042, 0.04000000000000000083, 0.05999999999999999778, 0.08000000000000000167, 0.1000000000000000194 ),
 .UNSPECIFIED. ) 
 CURVE ( )  GEOMETRIC_REPRESENTATION_ITEM ( )  RATIONAL_B_SPLINE_CURVE ( ( 1.000000000000000000, 0.9510565162951535312, 1.000000000000000000, 0.9510565162951535312, 1.000000000000000000, 0.9510565162951535312, 1.000000000000000000, 0.9510565162951535312, 1.000000000000000000, 0.9510565162951535312, 1.000000000000000000 ) ) 
 REPRESENTATION_ITEM ( '' )  );
#7062=CARTESIAN_POINT ( 'NONE',  ( 105.6631189606246153, 114.1144967660473242, -55.29999999453764303 ) ) ;
#7077=CARTESIAN_POINT ( 'NONE',  ( 108.0825317500000011, 110.0000000000000000, -48.87499999726882294 ) ) ;
#7107=CARTESIAN_POINT ( 'NONE',  ( 99.99999999999997158, 101.5015231886685854, -49.12499999726882294 ) ) ;
#7125=DIRECTION ( 'NONE',  ( -0.8660254037844392627, -0.000000000000000000, 0.4999999999999987788 ) ) ;
#7132=CARTESIAN_POINT ( 'NONE',  ( 104.9952793366501567, 116.8754121666685393, -52.32499999726881867 ) ) ;
#7157=FACE_OUTER_BOUND ( 'NONE', #21496, .T. ) ;
#7167=CARTESIAN_POINT ( 'NONE',  ( 99.99999999999997158, 118.4984768113314004, -46.37499999726880873 ) ) ;
#7175=EDGE_LOOP ( 'NONE', ( #11411, #16309, #5568, #10498 ) ) ;
#7205=( BOUNDED_CURVE ( )  B_SPLINE_CURVE ( 2, ( #20992, #27409, #5608, #3322, #9587, #12267, #7444, #14274, #23272, #1473, #7872 ),
 .UNSPECIFIED., .F., .F. ) 
 B_SPLINE_CURVE_WITH_KNOTS ( ( 3, 2, 2, 2, 2, 3 ),
 ( 0.4999999999999996669, 0.5199999999999996847, 0.5399999999999998135, 0.5599999999999998312, 0.5799999999999998490, 0.5999999999999998668 ),
 .UNSPECIFIED. ) 
 CURVE ( )  GEOMETRIC_REPRESENTATION_ITEM ( )  RATIONAL_B_SPLINE_CURVE ( ( 1.000000000000000888, 0.9510565162951527540, 1.000000000000000000, 0.9510565162951535312, 1.000000000000000000, 0.9510565162951535312, 1.000000000000000000, 0.9510565162951535312, 1.000000000000000000, 0.9510565162951537532, 0.9999999999999997780 ) ) 
 REPRESENTATION_ITEM ( '' )  );
#7214=CIRCLE ( 'NONE', #24976, 7.000000000000006217 ) ;
#7216=CARTESIAN_POINT ( 'NONE',  ( 99.99999999999997158, 101.5015231886685712, -51.37499999726882294 ) ) ;
#7228=CARTESIAN_POINT ( 'NONE',  ( 97.83688103937535629, 116.6573956140660897, -45.40000000000001279 ) ) ;
#7252=CARTESIAN_POINT ( 'NONE',  ( 108.0825317500000011, 110.0000000000000000, -46.62499999726882294 ) ) ;
#7279=VECTOR ( 'NONE', #27154, 1000.000000000000000 ) ;
#7287=CARTESIAN_POINT ( 'NONE',  ( 93.00000000000000000, 112.2744378736303332, -48.59999999453764019 ) ) ;
#7315=CARTESIAN_POINT ( 'NONE',  ( 91.91746824999997045, 112.6261737610028320, -51.97499999726882436 ) ) ;
#7323=VERTEX_POINT ( 'NONE', #5224 ) ;
#7344=CARTESIAN_POINT ( 'NONE',  ( 105.6631189606246153, 114.1144967660473242, -53.29999999453764303 ) ) ;
#7360=CARTESIAN_POINT ( 'NONE',  ( 95.00472066334981491, 116.8754121666685393, -54.17499999726882720 ) ) ;
#7366=CARTESIAN_POINT ( 'NONE',  ( 106.9999999999999716, 112.2744378736303759, -51.39999999453765156 ) ) ;
#7392=CARTESIAN_POINT ( 'NONE',  ( 94.33688103937535629, 105.8855032339526758, -54.80000000000001847 ) ) ;
#7444=CARTESIAN_POINT ( 'NONE',  ( 97.83688103937537051, 103.3426043859339103, -50.60000000000001563 ) ) ;
#7456=CARTESIAN_POINT ( 'NONE',  ( 99.99999999999997158, 101.5015231886685854, -51.37499999726882294 ) ) ;
#7488=CARTESIAN_POINT ( 'NONE',  ( 95.67376207875072680, 115.9545556584642867, -52.79999999453764303 ) ) ;
#7493=CARTESIAN_POINT ( 'NONE',  ( 94.33688103937534208, 114.1144967660473242, -51.20000000000000995 ) ) ;
#7506=CARTESIAN_POINT ( 'NONE',  ( 97.50236033167490746, 117.6869444889999841, -50.27499999726882152 ) ) ;
#7530=CARTESIAN_POINT ( 'NONE',  ( 106.5389055433250860, 114.7507929638356785, -54.67499999726882720 ) ) ;
#7539=CARTESIAN_POINT ( 'NONE',  ( 104.9952793366501709, 103.1245878333314323, -48.92499999726882010 ) ) ;
#7607=CARTESIAN_POINT ( 'NONE',  ( 97.50236033167490746, 102.3130555110000159, -47.47499999726881725 ) ) ;
#7649=MANIFOLD_SOLID_BREP ( 'Thread1', #14440 ) ;
#7654=CARTESIAN_POINT ( 'NONE',  ( 108.0825317500000011, 110.0000000000000000, -50.87499999726882294 ) ) ;
#7660=CARTESIAN_POINT ( 'NONE',  ( 107.0000000000000000, 110.0000000000000000, -51.49999999453763877 ) ) ;
#7676=CARTESIAN_POINT ( 'NONE',  ( 102.4976396683250783, 102.3130555110000159, -55.27499999726882152 ) ) ;
#7683=AXIS2_PLACEMENT_3D ( 'NONE', #21070, #3688, #12481 ) ;
#7685=CARTESIAN_POINT ( 'NONE',  ( 99.99999999999997158, 118.4984768113314004, -48.12499999726881583 ) ) ;
#7713=CARTESIAN_POINT ( 'NONE',  ( 106.5389055433250860, 105.2492070361643215, -52.82499999726881867 ) ) ;
#7719=ORIENTED_EDGE ( 'NONE', *, *, #9595, .T. ) ;
#7741=ORIENTED_EDGE ( 'NONE', *, *, #11083, .T. ) ;
#7746=LINE ( 'NONE', #18853, #7279 ) ;
#7747=CARTESIAN_POINT ( 'NONE',  ( 99.99999999999997158, 101.5015231886685854, -49.37499999726882294 ) ) ;
#7777=LINE ( 'NONE', #12310, #19119 ) ;
#7796=CARTESIAN_POINT ( 'NONE',  ( 91.91746824999998466, 110.0000000000000000, -53.87499999726882294 ) ) ;
#7805=DIRECTION ( 'NONE',  ( 5.782411586589358625E-17, -0.000000000000000000, 1.000000000000000000 ) ) ;
#7816=CARTESIAN_POINT ( 'NONE',  ( 107.0000000000000000, 107.7255621263696668, -46.10000000000000142 ) ) ;
#7820=CARTESIAN_POINT ( 'NONE',  ( 97.50236033167490746, 102.3130555110000159, -53.47499999726882436 ) ) ;
#7827=CARTESIAN_POINT ( 'NONE',  ( 91.91746824999997045, 107.3738262389971538, -51.52499999726882152 ) ) ;
#7872=CARTESIAN_POINT ( 'NONE',  ( 92.99999999999998579, 110.0000000000000000, -51.00000000000000711 ) ) ;
#7884=CARTESIAN_POINT ( 'NONE',  ( 95.00472066334982912, 103.1245878333314323, -55.57499999726881157 ) ) ;
#7893=ORIENTED_EDGE ( 'NONE', *, *, #8047, .F. ) ;
#7914=CARTESIAN_POINT ( 'NONE',  ( 104.9952793366501709, 116.8754121666685393, -46.32499999726881867 ) ) ;
#7935=CARTESIAN_POINT ( 'NONE',  ( 102.1631189606246153, 116.6573956140660897, -51.09999999453764019 ) ) ;
#7936=VECTOR ( 'NONE', #24823, 1000.000000000000000 ) ;
#7951=CARTESIAN_POINT ( 'NONE',  ( 97.83688103937537051, 103.3426043859339103, -50.09999999453764019 ) ) ;
#7959=VECTOR ( 'NONE', #3521, 1000.000000000000000 ) ;
#7960=CARTESIAN_POINT ( 'NONE',  ( 95.00472066334982912, 103.1245878333314323, -51.32499999726880446 ) ) ;
#8047=EDGE_CURVE ( 'NONE', #12248, #8859, #9084, .T. ) ;
#8051=CARTESIAN_POINT ( 'NONE',  ( 97.50236033167490746, 102.3130555110000159, -49.22499999726882436 ) ) ;
#8090=CARTESIAN_POINT ( 'NONE',  ( 102.1631189606246153, 116.6573956140660897, -53.09999999453764019 ) ) ;
#8093=CARTESIAN_POINT ( 'NONE',  ( 94.33688103937535629, 105.8855032339526758, -52.29999999453764303 ) ) ;
#8100=CARTESIAN_POINT ( 'NONE',  ( 106.5389055433250860, 114.7507929638356785, -54.42499999726882720 ) ) ;
#8129=ADVANCED_FACE ( 'NONE', ( #26797 ), #11511, .T. ) ;
#8191=FACE_BOUND ( 'NONE', #20868, .T. ) ;
#8215=CARTESIAN_POINT ( 'NONE',  ( 99.99999999999997158, 102.6397644303321215, -49.99999999453764588 ) ) ;
#8226=CARTESIAN_POINT ( 'NONE',  ( 107.0000000000000000, 112.2744378736303332, -51.39999999453764445 ) ) ;
#8245=EDGE_CURVE ( 'NONE', #24786, #789, #4358, .T. ) ;
#8248=CARTESIAN_POINT ( 'NONE',  ( 99.99999999999997158, 102.6397644303321215, -48.50000000000000711 ) ) ;
#8292=CARTESIAN_POINT ( 'NONE',  ( 102.4976396683250783, 102.3130555110000159, -47.27499999726882152 ) ) ;
#8294=( LENGTH_UNIT ( ) NAMED_UNIT ( * ) SI_UNIT ( .MILLI., .METRE. ) );
#8299=CARTESIAN_POINT ( 'NONE',  ( 104.9952793366501709, 116.8754121666685393, -54.57499999726882578 ) ) ;
#8317=ORIENTED_EDGE ( 'NONE', *, *, #8370, .F. ) ;
#8320=FILL_AREA_STYLE ('',( #8741 ) ) ;
#8329=CARTESIAN_POINT ( 'NONE',  ( 93.46109445667489979, 114.7507929638356785, -45.82499999726881867 ) ) ;
#8362=CARTESIAN_POINT ( 'NONE',  ( 107.0000000000000000, 110.0000000000000000, -145.0000000000000284 ) ) ;
#8366=CARTESIAN_POINT ( 'NONE',  ( 94.33688103937535629, 105.8855032339526758, -52.29999999453764303 ) ) ;
#8370=EDGE_CURVE ( 'NONE', #12194, #15376, #16920, .T. ) ;
#8375=CARTESIAN_POINT ( 'NONE',  ( 104.9952793366501709, 116.8754121666685393, -52.32499999726881867 ) ) ;
#8381=( BOUNDED_SURFACE ( )  B_SPLINE_SURFACE ( 1, 2, ( 
 ( #16983, #21700, #17120, #4171, #2033, #10701, #6440, #10566, #27838, #21559, #21421, #15110, #4588, #4031, #8292, #12968, #23830, #33, #2175, #1900, #2320, #13105, #17408, #25824, #2456, #19552, #11118, #4451, #8858, #6164, #14830, #12832, #10837, #19275, #4311, #13248, #27973, #23554, #26107, #6572, #15255, #23973, #8431, #10977, #21844, #19689, #6298, #14975, #176, #23694, #17549, #26253, #8576, #17266, #25967, #6713, #15399, #24112, #21980, #22939, #14221, #24392, #11796, #19832, #18373, #24926, #4734, #20797, #9811, #6854, #18517, #13394, #9142, #15543, #3402, #27078, #7820, #26399, #5412, #25069, #3269, #9670, #12072, #11937, #20659, #1277, #1144, #24252, #7530, #23074, #3130, #317, #5556, #27361, #7676, #20519, #27222, #4880, #13544, #26540, #16368 ),
 ( #22266, #1001, #9942, #6996, #9005, #16226, #22122, #18657, #15690, #16512, #14080, #3550, #22800, #25205, #5691, #14358, #17697, #2601, #11262, #19983, #461, #17835, #18789, #23761, #27768, #12767, #19340, #21071, #10351, #3822, #6099, #1559, #15044, #20934, #23485, #23626, #7951, #14905, #12626, #4102, #21209, #3966, #25344, #5829, #10077, #25901, #27905, #25484, #28044, #8226, #8511, #14766, #23214, #19060, #25755, #14497, #5962, #12482, #8366, #18922, #1418, #14630, #3689, #10496, #27630, #19203, #8090, #12207, #16785, #23349, #1694, #21485, #17194, #10634, #6371, #25616, #1966, #16916, #27496, #16649, #21352, #12353, #10212, #1832, #17051, #6237, #26325, #13036, #7062, #12897, #15470, #15618, #28180, #6924, #4662, #24320, #13177, #24184, #17339, #26036, #2103 ) ),
 .UNSPECIFIED., .F., .F., .F. ) 
 B_SPLINE_SURFACE_WITH_KNOTS ( ( 2, 2 ),
 ( 3, 2, 2, 2, 2, 2, 2, 2, 2, 2, 2, 2, 2, 2, 2, 2, 2, 2, 2, 2, 2, 2, 2, 2, 2, 2, 2, 2, 2, 2, 2, 2, 2, 2, 2, 2, 2, 2, 2, 2, 2, 2, 2, 2, 2, 2, 2, 2, 2, 2, 3 ),
 ( 0.000000000000000000, 1.000000000000000000 ),
 ( 0.000000000000000000, 0.02000000000000000042, 0.04000000000000000083, 0.05999999999999999778, 0.08000000000000000167, 0.1000000000000000056, 0.1199999999999999956, 0.1400000000000000133, 0.1600000000000000033, 0.1799999999999999933, 0.2000000000000000111, 0.2200000000000000011, 0.2399999999999999911, 0.2600000000000000089, 0.2800000000000000266, 0.2999999999999999889, 0.3200000000000000067, 0.3400000000000000244, 0.3599999999999999867, 0.3800000000000000044, 0.4000000000000000222, 0.4199999999999999845, 0.4400000000000000022, 0.4600000000000000200, 0.4799999999999999822, 0.5000000000000000000, 0.5200000000000000178, 0.5400000000000000355, 0.5600000000000000533, 0.5799999999999999600, 0.5999999999999999778, 0.6199999999999999956, 0.6400000000000000133, 0.6600000000000000311, 0.6800000000000000488, 0.6999999999999999556, 0.7199999999999999734, 0.7399999999999999911, 0.7600000000000000089, 0.7800000000000000266, 0.8000000000000000444, 0.8199999999999999512, 0.8399999999999999689, 0.8599999999999999867, 0.8800000000000000044, 0.9000000000000000222, 0.9200000000000000400, 0.9399999999999999467, 0.9599999999999999645, 0.9799999999999999822, 1.000000000000000000 ),
 .UNSPECIFIED. ) 
 GEOMETRIC_REPRESENTATION_ITEM ( )  RATIONAL_B_SPLINE_SURFACE ( (
 ( 1.000000000000000000, 0.9510565162951535312, 1.000000000000000000, 0.9510565162951535312, 1.000000000000000000, 0.9510565162951535312, 1.000000000000000000, 0.9510565162951535312, 1.000000000000000000, 0.9510565162951535312, 1.000000000000000000, 0.9510565162951535312, 1.000000000000000000, 0.9510565162951535312, 1.000000000000000000, 0.9510565162951535312, 1.000000000000000000, 0.9510565162951535312, 1.000000000000000000, 0.9510565162951535312, 1.000000000000000000, 0.9510565162951535312, 1.000000000000000000, 0.9510565162951535312, 1.000000000000000000, 0.9510565162951535312, 1.000000000000000000, 0.9510565162951535312, 1.000000000000000000, 0.9510565162951535312, 1.000000000000000000, 0.9510565162951535312, 1.000000000000000000, 0.9510565162951535312, 1.000000000000000000, 0.9510565162951535312, 1.000000000000000000, 0.9510565162951535312, 1.000000000000000000, 0.9510565162951535312, 1.000000000000000000, 0.9510565162951535312, 1.000000000000000000, 0.9510565162951535312, 1.000000000000000000, 0.9510565162951535312, 1.000000000000000000, 0.9510565162951535312, 1.000000000000000000, 0.9510565162951535312, 1.000000000000000000, 0.9510565162951535312, 1.000000000000000000, 0.9510565162951535312, 1.000000000000000000, 0.9510565162951535312, 1.000000000000000000, 0.9510565162951535312, 1.000000000000000000, 0.9510565162951535312, 1.000000000000000000, 0.9510565162951535312, 1.000000000000000000, 0.9510565162951535312, 1.000000000000000000, 0.9510565162951535312, 1.000000000000000000, 0.9510565162951535312, 1.000000000000000000, 0.9510565162951535312, 1.000000000000000000, 0.9510565162951535312, 1.000000000000000000, 0.9510565162951535312, 1.000000000000000000, 0.9510565162951535312, 1.000000000000000000, 0.9510565162951535312, 1.000000000000000000, 0.9510565162951535312, 1.000000000000000000, 0.9510565162951535312, 1.000000000000000000, 0.9510565162951535312, 1.000000000000000000, 0.9510565162951535312, 1.000000000000000000, 0.9510565162951535312, 1.000000000000000000, 0.9510565162951535312, 1.000000000000000000, 0.9510565162951535312, 1.000000000000000000, 0.9510565162951535312, 1.000000000000000000, 0.9510565162951535312, 1.000000000000000000, 0.9510565162951535312, 1.000000000000000000, 0.9510565162951535312, 1.000000000000000000),
 ( 1.000000000000000000, 0.9510565162951535312, 1.000000000000000000, 0.9510565162951535312, 1.000000000000000000, 0.9510565162951535312, 1.000000000000000000, 0.9510565162951535312, 1.000000000000000000, 0.9510565162951535312, 1.000000000000000000, 0.9510565162951535312, 1.000000000000000000, 0.9510565162951535312, 1.000000000000000000, 0.9510565162951535312, 1.000000000000000000, 0.9510565162951535312, 1.000000000000000000, 0.9510565162951535312, 1.000000000000000000, 0.9510565162951535312, 1.000000000000000000, 0.9510565162951535312, 1.000000000000000000, 0.9510565162951535312, 1.000000000000000000, 0.9510565162951535312, 1.000000000000000000, 0.9510565162951535312, 1.000000000000000000, 0.9510565162951535312, 1.000000000000000000, 0.9510565162951535312, 1.000000000000000000, 0.9510565162951535312, 1.000000000000000000, 0.9510565162951535312, 1.000000000000000000, 0.9510565162951535312, 1.000000000000000000, 0.9510565162951535312, 1.000000000000000000, 0.9510565162951535312, 1.000000000000000000, 0.9510565162951535312, 1.000000000000000000, 0.9510565162951535312, 1.000000000000000000, 0.9510565162951535312, 1.000000000000000000, 0.9510565162951535312, 1.000000000000000000, 0.9510565162951535312, 1.000000000000000000, 0.9510565162951535312, 1.000000000000000000, 0.9510565162951535312, 1.000000000000000000, 0.9510565162951535312, 1.000000000000000000, 0.9510565162951535312, 1.000000000000000000, 0.9510565162951535312, 1.000000000000000000, 0.9510565162951535312, 1.000000000000000000, 0.9510565162951535312, 1.000000000000000000, 0.9510565162951535312, 1.000000000000000000, 0.9510565162951535312, 1.000000000000000000, 0.9510565162951535312, 1.000000000000000000, 0.9510565162951535312, 1.000000000000000000, 0.9510565162951535312, 1.000000000000000000, 0.9510565162951535312, 1.000000000000000000, 0.9510565162951535312, 1.000000000000000000, 0.9510565162951535312, 1.000000000000000000, 0.9510565162951535312, 1.000000000000000000, 0.9510565162951535312, 1.000000000000000000, 0.9510565162951535312, 1.000000000000000000, 0.9510565162951535312, 1.000000000000000000, 0.9510565162951535312, 1.000000000000000000, 0.9510565162951535312, 1.000000000000000000, 0.9510565162951535312, 1.000000000000000000, 0.9510565162951535312, 1.000000000000000000) ) ) 
 REPRESENTATION_ITEM ( '' )  SURFACE ( )  );
#8398=ORIENTED_EDGE ( 'NONE', *, *, #5495, .T. ) ;
#8405=ORIENTED_EDGE ( 'NONE', *, *, #14283, .F. ) ;
#8429=CARTESIAN_POINT ( 'NONE',  ( 95.00472066334981491, 116.8754121666685393, -45.92499999726882720 ) ) ;
#8431=CARTESIAN_POINT ( 'NONE',  ( 93.46109445667489979, 114.7507929638356785, -50.07499999726882578 ) ) ;
#8433=FILL_AREA_STYLE ('',( #25415 ) ) ;
#8437=CARTESIAN_POINT ( 'NONE',  ( 91.91746824999997045, 112.6261737610028320, -53.97499999726881725 ) ) ;
#8460=( NAMED_UNIT ( * ) PLANE_ANGLE_UNIT ( ) SI_UNIT ( $, .RADIAN. ) );
#8472=CARTESIAN_POINT ( 'NONE',  ( 95.00472066334982912, 116.8754121666685393, -47.92499999726882010 ) ) ;
#8511=CARTESIAN_POINT ( 'NONE',  ( 107.0000000000000000, 110.0000000000000000, -51.49999999453763877 ) ) ;
#8547=CARTESIAN_POINT ( 'NONE',  ( 95.67376207875069838, 115.9545556584642867, -45.30000000000000426 ) ) ;
#8551=LINE ( 'NONE', #17383, #21293 ) ;
#8568=DIRECTION ( 'NONE',  ( 1.000000000000000000, 0.000000000000000000, 0.000000000000000000 ) ) ;
#8571=MECHANICAL_DESIGN_GEOMETRIC_PRESENTATION_REPRESENTATION('',(#5458),#14919);
#8574=CARTESIAN_POINT ( 'NONE',  ( 99.99999999999997158, 118.4984768113314146, -46.12499999726881583 ) ) ;
#8576=CARTESIAN_POINT ( 'NONE',  ( 106.5389055433250860, 105.2492070361643215, -51.07499999726882578 ) ) ;
#8591=DIRECTION ( 'NONE',  ( 1.000000000000000000, 0.000000000000000000, 0.000000000000000000 ) ) ;
#8600=EDGE_CURVE ( 'NONE', #3776, #22871, #25662, .T. ) ;
#8612=CARTESIAN_POINT ( 'NONE',  ( 102.4976396683250783, 117.6869444889999841, -54.22499999726881725 ) ) ;
#8635=CARTESIAN_POINT ( 'NONE',  ( 0.000000000000000000, 0.000000000000000000, 0.000000000000000000 ) ) ;
#8661=CARTESIAN_POINT ( 'NONE',  ( 91.91746824999998466, 110.0000000000000000, -47.87499999726882294 ) ) ;
#8690=CARTESIAN_POINT ( 'NONE',  ( 94.33688103937535629, 105.8855032339526758, -50.80000000000001137 ) ) ;
#8711=CARTESIAN_POINT ( 'NONE',  ( 99.99999999999998579, 110.0000000000000000, -145.0000000000000284 ) ) ;
#8713=CARTESIAN_POINT ( 'NONE',  ( 95.00472066334981491, 103.1245878333314465, -49.32499999726881867 ) ) ;
#8739=ORIENTED_EDGE ( 'NONE', *, *, #6071, .F. ) ;
#8741=FILL_AREA_STYLE_COLOUR ( '', #26386 ) ;
#8744=PRODUCT_DEFINITION_SHAPE ( 'NONE', 'NONE',  #22512 ) ;
#8751=CARTESIAN_POINT ( 'NONE',  ( 108.0825317499999869, 107.3738262389971538, -50.72499999726881015 ) ) ;
#8787=CARTESIAN_POINT ( 'NONE',  ( 107.0000000000000000, 110.0000000000000000, -50.00000000000000711 ) ) ;
#8825=ORIENTED_EDGE ( 'NONE', *, *, #956, .F. ) ;
#8831=CARTESIAN_POINT ( 'NONE',  ( 97.83688103937537051, 103.3426043859339103, -52.60000000000001563 ) ) ;
#8844=EDGE_LOOP ( 'NONE', ( #6752, #1772, #10137, #21728 ) ) ;
#8856=CARTESIAN_POINT ( 'NONE',  ( 108.0825317499999869, 112.6261737610028320, -52.52499999726882152 ) ) ;
#8858=CARTESIAN_POINT ( 'NONE',  ( 106.5389055433250860, 114.7507929638356785, -48.67499999726882010 ) ) ;
#8859=VERTEX_POINT ( 'NONE', #25035 ) ;
#8894=CARTESIAN_POINT ( 'NONE',  ( 91.91746824999997045, 107.3738262389971538, -51.52499999726882152 ) ) ;
#8895=VERTEX_POINT ( 'NONE', #18621 ) ;
#8926=CYLINDRICAL_SURFACE ( 'NONE', #16661, 5.000000000000004441 ) ;
#8941=CARTESIAN_POINT ( 'NONE',  ( 108.0825317499999869, 112.6261737610028320, -48.77499999726882152 ) ) ;
#8974=CARTESIAN_POINT ( 'NONE',  ( 93.00000000000000000, 112.2744378736303332, -53.10000000000000142 ) ) ;
#9002=CARTESIAN_POINT ( 'NONE',  ( 104.9952793366501567, 103.1245878333314465, -50.92499999726882010 ) ) ;
#9005=CARTESIAN_POINT ( 'NONE',  ( 97.83688103937535629, 116.6573956140660897, -46.89999999453763735 ) ) ;
#9011=ORIENTED_EDGE ( 'NONE', *, *, #10160, .F. ) ;
#9015=VERTEX_POINT ( 'NONE', #11359 ) ;
#9021=CARTESIAN_POINT ( 'NONE',  ( 99.99999999999998579, 110.0000000000000000, -145.0000000000000284 ) ) ;
#9038=CARTESIAN_POINT ( 'NONE',  ( 91.91746824999997045, 107.3738262389971538, -55.52499999726882862 ) ) ;
#9039=VECTOR ( 'NONE', #12896, 1000.000000000000000 ) ;
#9046=PLANE ( 'NONE',  #23429 ) ;
#9071=CARTESIAN_POINT ( 'NONE',  ( 105.6631189606246153, 114.1144967660473242, -55.29999999453764303 ) ) ;
#9084=CIRCLE ( 'NONE', #6352, 7.000000000000006217 ) ;
#9086=CARTESIAN_POINT ( 'NONE',  ( 108.0825317500000011, 110.0000000000000000, -46.87499999726882294 ) ) ;
#9096=CARTESIAN_POINT ( 'NONE',  ( 104.3262379212492448, 115.9545556584642867, -45.70000000000000995 ) ) ;
#9115=CARTESIAN_POINT ( 'NONE',  ( 102.1631189606246295, 103.3426043859339103, -48.40000000000001279 ) ) ;
#9140=CARTESIAN_POINT ( 'NONE',  ( 102.4976396683250783, 117.6869444889999841, -48.22499999726881725 ) ) ;
#9142=CARTESIAN_POINT ( 'NONE',  ( 106.5389055433250860, 105.2492070361643215, -53.07499999726881867 ) ) ;
#9179=CARTESIAN_POINT ( 'NONE',  ( 95.00472066334982912, 103.1245878333314323, -51.32499999726880446 ) ) ;
#9226=CARTESIAN_POINT ( 'NONE',  ( 91.91746824999998466, 110.0000000000000000, -45.87499999726882294 ) ) ;
#9235=LINE ( 'NONE', #17927, #16953 ) ;
#9251=ORIENTED_EDGE ( 'NONE', *, *, #11405, .T. ) ;
#9257=CARTESIAN_POINT ( 'NONE',  ( 94.33688103937534208, 114.1144967660473242, -51.20000000000000995 ) ) ;
#9272=DIRECTION ( 'NONE',  ( 1.000000000000000000, 0.000000000000000000, 0.000000000000000000 ) ) ;
#9279=CARTESIAN_POINT ( 'NONE',  ( 91.91746824999997045, 107.3738262389971680, -51.52499999726882152 ) ) ;
#9292=DIRECTION ( 'NONE',  ( -5.782411586589357392E-17, 0.000000000000000000, -1.000000000000000000 ) ) ;
#9313=CARTESIAN_POINT ( 'NONE',  ( 106.5389055433250860, 114.7507929638356785, -50.67499999726882010 ) ) ;
#9314=ORIENTED_EDGE ( 'NONE', *, *, #13713, .F. ) ;
#9332=EDGE_CURVE ( 'NONE', #24121, #1428, #17661, .T. ) ;
#9363=CARTESIAN_POINT ( 'NONE',  ( 108.0825317499999869, 112.6261737610028320, -50.77499999726882152 ) ) ;
#9368=CARTESIAN_POINT ( 'NONE',  ( 92.99999999999998579, 110.0000000000000000, -50.49999999453763877 ) ) ;
#9393=CARTESIAN_POINT ( 'NONE',  ( 91.91746824999997045, 112.6261737610028320, -49.72499999726881725 ) ) ;
#9418=CARTESIAN_POINT ( 'NONE',  ( 95.00472066334981491, 103.1245878333314465, -55.32499999726882578 ) ) ;
#9426=CARTESIAN_POINT ( 'NONE',  ( 107.0000000000000000, 112.2744378736303190, -49.39999999453763735 ) ) ;
#9434=CARTESIAN_POINT ( 'NONE',  ( 94.33688103937534208, 114.1144967660473242, -53.20000000000000995 ) ) ;
#9455=CARTESIAN_POINT ( 'NONE',  ( 95.00472066334982912, 103.1245878333314323, -51.57499999726880446 ) ) ;
#9503=LINE ( 'NONE', #18204, #4340 ) ;
#9505=CARTESIAN_POINT ( 'NONE',  ( 102.4976396683250783, 117.6869444889999841, -50.47499999726882436 ) ) ;
#9536=CARTESIAN_POINT ( 'NONE',  ( 102.1631189606246153, 116.6573956140660897, -47.60000000000000853 ) ) ;
#9540=CARTESIAN_POINT ( 'NONE',  ( 107.0000000000000000, 107.7255621263696668, -54.10000000000000853 ) ) ;
#9568=CARTESIAN_POINT ( 'NONE',  ( 92.99999999999998579, 110.0000000000000000, -45.74999999726882294 ) ) ;
#9571=VERTEX_POINT ( 'NONE', #19332 ) ;
#9587=CARTESIAN_POINT ( 'NONE',  ( 102.1631189606246295, 103.3426043859339103, -50.40000000000001279 ) ) ;
#9593=EDGE_LOOP ( 'NONE', ( #5358, #23086, #5501, #7741 ) ) ;
#9595=EDGE_CURVE ( 'NONE', #2581, #23665, #23753, .T. ) ;
#9599=CARTESIAN_POINT ( 'NONE',  ( 104.9952793366501709, 116.8754121666685393, -50.57499999726882578 ) ) ;
#9634=CARTESIAN_POINT ( 'NONE',  ( 95.67376207875072680, 115.9545556584642867, -51.30000000000000426 ) ) ;
#9646=CARTESIAN_POINT ( 'NONE',  ( 106.5389055433250860, 114.7507929638356785, -52.67499999726882010 ) ) ;
#9652=CARTESIAN_POINT ( 'NONE',  ( 92.99999999999997158, 112.2744378736302906, -50.59999999453763309 ) ) ;
#9670=CARTESIAN_POINT ( 'NONE',  ( 91.91746824999997045, 112.6261737610028320, -53.97499999726881725 ) ) ;
#9680=CARTESIAN_POINT ( 'NONE',  ( 104.9952793366501709, 116.8754121666685393, -48.32499999726881867 ) ) ;
#9716=ORIENTED_EDGE ( 'NONE', *, *, #11787, .F. ) ;
#9740=CARTESIAN_POINT ( 'NONE',  ( 104.9952793366501709, 116.8754121666685393, -48.57499999726881867 ) ) ;
#9744=CARTESIAN_POINT ( 'NONE',  ( 91.91746824999998466, 110.0000000000000000, -55.74999999726882294 ) ) ;
#9750=CARTESIAN_POINT ( 'NONE',  ( 99.99999999999998579, 110.0000000000000000, -145.0000000000000284 ) ) ;
#9786=CARTESIAN_POINT ( 'NONE',  ( 104.9952793366501567, 116.8754121666685393, -54.57499999726882578 ) ) ;
#9792=CARTESIAN_POINT ( 'NONE',  ( 105.6631189606246295, 105.8855032339526758, -52.20000000000000995 ) ) ;
#9811=CARTESIAN_POINT ( 'NONE',  ( 106.5389055433250860, 114.7507929638356785, -52.67499999726882010 ) ) ;
#9819=CARTESIAN_POINT ( 'NONE',  ( 104.9952793366501709, 103.1245878333314323, -46.92499999726882010 ) ) ;
#9868=CARTESIAN_POINT ( 'NONE',  ( 105.0000000000000000, 110.0000000000000000, -145.0000000000000284 ) ) ;
#9879=CARTESIAN_POINT ( 'NONE',  ( 104.9952793366501709, 103.1245878333314323, -47.17499999726881299 ) ) ;
#9917=CARTESIAN_POINT ( 'NONE',  ( 95.00472066334981491, 103.1245878333314465, -53.57499999726881157 ) ) ;
#9934=CARTESIAN_POINT ( 'NONE',  ( 99.99999999999998579, 110.0000000000000000, -45.00000000000000711 ) ) ;
#9942=CARTESIAN_POINT ( 'NONE',  ( 94.33688103937534208, 114.1144967660473242, -46.69999999453764161 ) ) ;
#9953=CARTESIAN_POINT ( 'NONE',  ( 108.0825317500000011, 110.0000000000000000, -48.62499999726882294 ) ) ;
#9984=ADVANCED_FACE ( 'NONE', ( #14496 ), #27495, .T. ) ;
#10000=CARTESIAN_POINT ( 'NONE',  ( 99.99999999999998579, 110.0000000000000000, -145.0000000000000284 ) ) ;
#10014=CARTESIAN_POINT ( 'NONE',  ( 93.46109445667489979, 105.2492070361643215, -53.67499999726882720 ) ) ;
#10035=CARTESIAN_POINT ( 'NONE',  ( 92.99999999999998579, 110.0000000000000000, -47.00000000000001421 ) ) ;
#10041=CARTESIAN_POINT ( 'NONE',  ( 108.0825317500000011, 110.0000000000000000, -48.62499999726882294 ) ) ;
#10044=PRODUCT_DEFINITION_CONTEXT ( 'detailed design', #24064, 'design' ) ;
#10077=CARTESIAN_POINT ( 'NONE',  ( 97.83688103937535629, 116.6573956140660897, -50.89999999453764445 ) ) ;
#10080=CARTESIAN_POINT ( 'NONE',  ( 107.0000000000000142, 107.7255621263696952, -51.59999999453763309 ) ) ;
#10137=ORIENTED_EDGE ( 'NONE', *, *, #16294, .T. ) ;
#10138=( NAMED_UNIT ( * ) SI_UNIT ( $, .STERADIAN. ) SOLID_ANGLE_UNIT ( ) );
#10139=CARTESIAN_POINT ( 'NONE',  ( 97.83688103937537051, 103.3426043859339103, -54.09999999453764019 ) ) ;
#10160=EDGE_CURVE ( 'NONE', #8859, #12194, #21627, .T. ) ;
#10171=CARTESIAN_POINT ( 'NONE',  ( 99.99999999999997158, 101.5015231886685854, -47.12499999726882294 ) ) ;
#10203=EDGE_CURVE ( 'NONE', #21009, #9571, #388, .T. ) ;
#10212=CARTESIAN_POINT ( 'NONE',  ( 94.33688103937534208, 114.1144967660473242, -54.69999999453764161 ) ) ;
#10221=CARTESIAN_POINT ( 'NONE',  ( 99.99999999999997158, 101.5015231886685854, -51.12499999726882294 ) ) ;
#10250=AXIS2_PLACEMENT_3D ( 'NONE', #15263, #21431, #12560 ) ;
#10284=CARTESIAN_POINT ( 'NONE',  ( 97.50236033167490746, 117.6869444889999841, -54.27499999726882862 ) ) ;
#10302=( LENGTH_UNIT ( ) NAMED_UNIT ( * ) SI_UNIT ( .MILLI., .METRE. ) );
#10351=CARTESIAN_POINT ( 'NONE',  ( 105.6631189606246153, 114.1144967660473242, -49.29999999453763593 ) ) ;
#10360=CARTESIAN_POINT ( 'NONE',  ( 91.91746824999997045, 107.3738262389971538, -55.52499999726882862 ) ) ;
#10369=( BOUNDED_CURVE ( )  B_SPLINE_CURVE ( 2, ( #11050, #15759, #15328, #21628, #17767, #11330, #19906, #4519, #11187, #17475, #8787 ),
 .UNSPECIFIED., .F., .F. ) 
 B_SPLINE_CURVE_WITH_KNOTS ( ( 3, 2, 2, 2, 2, 3 ),
 ( 0.4000000000000003553, 0.4200000000000002065, 0.4400000000000000577, 0.4599999999999999645, 0.4799999999999997602, 0.4999999999999996669 ),
 .UNSPECIFIED. ) 
 CURVE ( )  GEOMETRIC_REPRESENTATION_ITEM ( )  RATIONAL_B_SPLINE_CURVE ( ( 0.9999999999999992228, 0.9510565162951543083, 1.000000000000000000, 0.9510565162951535312, 1.000000000000000000, 0.9510565162951535312, 1.000000000000000000, 0.9510565162951535312, 1.000000000000000000, 0.9510565162951543083, 0.9999999999999992228 ) ) 
 REPRESENTATION_ITEM ( '' )  );
#10396=CARTESIAN_POINT ( 'NONE',  ( 105.6631189606246295, 105.8855032339526758, -46.20000000000000995 ) ) ;
#10426=CARTESIAN_POINT ( 'NONE',  ( 92.99999999999998579, 110.0000000000000000, -54.49999999453763877 ) ) ;
#10429=CARTESIAN_POINT ( 'NONE',  ( 108.0825317499999869, 112.6261737610028320, -52.77499999726883573 ) ) ;
#10431=( GEOMETRIC_REPRESENTATION_CONTEXT ( 3 ) GLOBAL_UNCERTAINTY_ASSIGNED_CONTEXT ( ( #16613 ) ) GLOBAL_UNIT_ASSIGNED_CONTEXT ( ( #16598, #8460, #23855 ) ) REPRESENTATION_CONTEXT ( 'NONE', 'WORKASPACE' ) );
#10446=ORIENTED_EDGE ( 'NONE', *, *, #15415, .F. ) ;
#10496=CARTESIAN_POINT ( 'NONE',  ( 95.67376207875069838, 115.9545556584642867, -52.79999999453764303 ) ) ;
#10498=ORIENTED_EDGE ( 'NONE', *, *, #5538, .T. ) ;
#10505=CARTESIAN_POINT ( 'NONE',  ( 99.99999999999997158, 118.4984768113314004, -50.12499999726881583 ) ) ;
#10507=ORIENTED_EDGE ( 'NONE', *, *, #118, .T. ) ;
#10536=ADVANCED_FACE ( 'NONE', ( #12312, #8191 ), #14729, .T. ) ;
#10537=CARTESIAN_POINT ( 'NONE',  ( 95.67376207875069838, 104.0454443415356991, -46.70000000000000284 ) ) ;
#10563=CARTESIAN_POINT ( 'NONE',  ( 93.46109445667489979, 114.7507929638356785, -45.82499999726881867 ) ) ;
#10566=CARTESIAN_POINT ( 'NONE',  ( 104.9952793366501709, 116.8754121666685393, -46.57499999726881157 ) ) ;
#10571=CARTESIAN_POINT ( 'NONE',  ( 99.99999999999997158, 101.5015231886685854, -53.37499999726883004 ) ) ;
#10600=CARTESIAN_POINT ( 'NONE',  ( 93.46109445667489979, 114.7507929638356785, -47.82499999726882578 ) ) ;
#10623=CARTESIAN_POINT ( 'NONE',  ( 95.67376207875072680, 104.0454443415356991, -50.19999999453764161 ) ) ;
#10634=CARTESIAN_POINT ( 'NONE',  ( 104.3262379212492448, 104.0454443415356991, -53.79999999453763593 ) ) ;
#10693=FACE_OUTER_BOUND ( 'NONE', #8844, .T. ) ;
#10701=CARTESIAN_POINT ( 'NONE',  ( 99.99999999999997158, 118.4984768113314004, -46.37499999726880873 ) ) ;
#10712=CARTESIAN_POINT ( 'NONE',  ( 107.0000000000000000, 110.0000000000000000, -48.00000000000001421 ) ) ;
#10737=CARTESIAN_POINT ( 'NONE',  ( 102.4976396683250783, 102.3130555110000159, -53.02499999726882862 ) ) ;
#10745=( BOUNDED_CURVE ( )  B_SPLINE_CURVE ( 2, ( #2822, #22781, #9792, #13769, #20639, #840, #3108, #24483, #17923, #18500, #26920 ),
 .UNSPECIFIED., .F., .F. ) 
 B_SPLINE_CURVE_WITH_KNOTS ( ( 3, 2, 2, 2, 2, 3 ),
 ( 0.6999999999999998446, 0.7199999999999998623, 0.7399999999999998801, 0.7600000000000000089, 0.7800000000000000266, 0.8000000000000000444 ),
 .UNSPECIFIED. ) 
 CURVE ( )  GEOMETRIC_REPRESENTATION_ITEM ( )  RATIONAL_B_SPLINE_CURVE ( ( 1.000000000000000222, 0.9510565162951533091, 1.000000000000000000, 0.9510565162951535312, 1.000000000000000000, 0.9510565162951535312, 1.000000000000000000, 0.9510565162951535312, 1.000000000000000000, 0.9510565162951535312, 1.000000000000000000 ) ) 
 REPRESENTATION_ITEM ( '' )  );
#10771=CARTESIAN_POINT ( 'NONE',  ( 102.1631189606246153, 116.6573956140660897, -55.09999999453764019 ) ) ;
#10809=CARTESIAN_POINT ( 'NONE',  ( 93.00000000000000000, 112.2744378736303332, -49.10000000000000853 ) ) ;
#10832=PRODUCT_DEFINITION_FORMATION_WITH_SPECIFIED_SOURCE ( 'ANY', '', #26282, .NOT_KNOWN. ) ;
#10835=CARTESIAN_POINT ( 'NONE',  ( 102.4976396683250783, 102.3130555110000159, -49.02499999726882152 ) ) ;
#10837=CARTESIAN_POINT ( 'NONE',  ( 106.5389055433250860, 105.2492070361643215, -49.07499999726882578 ) ) ;
#10849=VERTEX_POINT ( 'NONE', #25269 ) ;
#10864=PRESENTATION_STYLE_ASSIGNMENT (( #6056 ) ) ;
#10877=CARTESIAN_POINT ( 'NONE',  ( 99.99999999999997158, 118.4984768113314004, -50.12499999726881583 ) ) ;
#10885=EDGE_CURVE ( 'NONE', #12248, #15376, #7746, .T. ) ;
#10925=CARTESIAN_POINT ( 'NONE',  ( 106.5389055433250860, 105.2492070361643215, -49.07499999726882578 ) ) ;
#10952=CARTESIAN_POINT ( 'NONE',  ( 105.6631189606246295, 105.8855032339526758, -52.20000000000000995 ) ) ;
#10975=CARTESIAN_POINT ( 'NONE',  ( 97.50236033167490746, 117.6869444889999841, -52.02499999726882862 ) ) ;
#10977=CARTESIAN_POINT ( 'NONE',  ( 95.00472066334982912, 116.8754121666685393, -50.17499999726882010 ) ) ;
#11010=CARTESIAN_POINT ( 'NONE',  ( 108.0825317499999869, 112.6261737610028320, -50.52499999726881441 ) ) ;
#11050=CARTESIAN_POINT ( 'NONE',  ( 92.99999999999998579, 110.0000000000000000, -49.00000000000001421 ) ) ;
#11083=EDGE_CURVE ( 'NONE', #15376, #19908, #27247, .T. ) ;
#11093=CARTESIAN_POINT ( 'NONE',  ( 94.33688103937535629, 105.8855032339526758, -52.80000000000001137 ) ) ;
#11116=CARTESIAN_POINT ( 'NONE',  ( 99.99999999999997158, 118.4984768113314146, -50.12499999726882294 ) ) ;
#11118=CARTESIAN_POINT ( 'NONE',  ( 102.4976396683250783, 117.6869444889999841, -48.47499999726882436 ) ) ;
#11126=CARTESIAN_POINT ( 'NONE',  ( 97.83688103937535629, 116.6573956140660897, -48.89999999453763735 ) ) ;
#11151=CARTESIAN_POINT ( 'NONE',  ( 106.5389055433250860, 105.2492070361643215, -54.82499999726882578 ) ) ;
#11165=CARTESIAN_POINT ( 'NONE',  ( 92.99999999999998579, 110.0000000000000000, -53.00000000000001421 ) ) ;
#11184=ADVANCED_FACE ( 'NONE', ( #5153 ), #22828, .T. ) ;
#11187=CARTESIAN_POINT ( 'NONE',  ( 105.6631189606246153, 114.1144967660473242, -49.80000000000001137 ) ) ;
#11190=CARTESIAN_POINT ( 'NONE',  ( 92.99999999999995737, 112.2744378736303048, -51.10000000000000853 ) ) ;
#11205=CARTESIAN_POINT ( 'NONE',  ( 91.91746824999997045, 112.6261737610028320, -49.97499999726882436 ) ) ;
#11210=CARTESIAN_POINT ( 'NONE',  ( 107.0000000000000000, 107.7255621263696668, -47.59999999453764019 ) ) ;
#11235=CARTESIAN_POINT ( 'NONE',  ( 105.6631189606246153, 114.1144967660473242, -47.80000000000001137 ) ) ;
#11248=VERTEX_POINT ( 'NONE', #14789 ) ;
#11260=CARTESIAN_POINT ( 'NONE',  ( 108.0825317499999869, 112.6261737610028320, -48.52499999726882152 ) ) ;
#11262=CARTESIAN_POINT ( 'NONE',  ( 94.33688103937535629, 105.8855032339526758, -48.29999999453764303 ) ) ;
#11285=DIRECTION ( 'NONE',  ( 5.782411586589358625E-17, -0.000000000000000000, 1.000000000000000000 ) ) ;
#11295=CARTESIAN_POINT ( 'NONE',  ( 93.46109445667489979, 114.7507929638356785, -53.82499999726881867 ) ) ;
#11330=CARTESIAN_POINT ( 'NONE',  ( 99.99999999999997158, 117.3602355696678643, -49.50000000000001421 ) ) ;
#11352=CARTESIAN_POINT ( 'NONE',  ( 107.0000000000000000, 110.0000000000000000, -145.0000000000000284 ) ) ;
#11359=CARTESIAN_POINT ( 'NONE',  ( 92.99999999999998579, 110.0000000000000000, -48.49999999453763877 ) ) ;
#11378=CARTESIAN_POINT ( 'NONE',  ( 105.6631189606246295, 105.8855032339526758, -50.20000000000001705 ) ) ;
#11402=CARTESIAN_POINT ( 'NONE',  ( 107.0000000000000000, 110.0000000000000000, -54.00000000000001421 ) ) ;
#11403=CARTESIAN_POINT ( 'NONE',  ( 108.0825317500000011, 110.0000000000000000, -50.62499999726882294 ) ) ;
#11405=EDGE_CURVE ( 'NONE', #22871, #20179, #10745, .T. ) ;
#11411=ORIENTED_EDGE ( 'NONE', *, *, #1492, .F. ) ;
#11439=CARTESIAN_POINT ( 'NONE',  ( 102.4976396683250783, 117.6869444889999841, -46.47499999726882436 ) ) ;
#11477=CARTESIAN_POINT ( 'NONE',  ( 99.99999999999997158, 117.3602355696678643, -51.50000000000001421 ) ) ;
#11486=CARTESIAN_POINT ( 'NONE',  ( 108.0825317499999869, 112.6261737610028320, -46.77499999726882152 ) ) ;
#11511=CYLINDRICAL_SURFACE ( 'NONE', #12706, 7.000000000000006217 ) ;
#11517=CARTESIAN_POINT ( 'NONE',  ( 108.0825317499999869, 107.3738262389971538, -46.72499999726881015 ) ) ;
#11552=CARTESIAN_POINT ( 'NONE',  ( 92.99999999999998579, 110.0000000000000000, -48.49999999453763877 ) ) ;
#11578=CARTESIAN_POINT ( 'NONE',  ( 106.5389055433250860, 105.2492070361643215, -51.07499999726882578 ) ) ;
#11617=( BOUNDED_CURVE ( )  B_SPLINE_CURVE ( 2, ( #18478, #18334, #13610, #7488, #674, #20050, #18188, #26898, #7344, #5512, #11755 ),
 .UNSPECIFIED., .F., .F. ) 
 B_SPLINE_CURVE_WITH_KNOTS ( ( 3, 2, 2, 2, 2, 3 ),
 ( 0.5999999999999998668, 0.6199999999999998845, 0.6399999999999999023, 0.6599999999999999201, 0.6799999999999999378, 0.6999999999999998446 ),
 .UNSPECIFIED. ) 
 CURVE ( )  GEOMETRIC_REPRESENTATION_ITEM ( )  RATIONAL_B_SPLINE_CURVE ( ( 1.000000000000000222, 0.9510565162951533091, 1.000000000000000000, 0.9510565162951535312, 1.000000000000000000, 0.9510565162951535312, 1.000000000000000000, 0.9510565162951535312, 1.000000000000000000, 0.9510565162951537532, 0.9999999999999997780 ) ) 
 REPRESENTATION_ITEM ( '' )  );
#11627=CARTESIAN_POINT ( 'NONE',  ( 93.46109445667489979, 105.2492070361643215, -55.67499999726882720 ) ) ;
#11660=CARTESIAN_POINT ( 'NONE',  ( 91.91746824999997045, 107.3738262389971538, -49.52499999726881441 ) ) ;
#11666=EDGE_LOOP ( 'NONE', ( #6503, #4650, #3733, #22267 ) ) ;
#11684=CARTESIAN_POINT ( 'NONE',  ( 91.91746824999998466, 110.0000000000000000, -55.62499999726882294 ) ) ;
#11721=CARTESIAN_POINT ( 'NONE',  ( 93.46109445667489979, 105.2492070361643215, -51.67499999726882010 ) ) ;
#11732=CYLINDRICAL_SURFACE ( 'NONE', #5629, 7.000000000000006217 ) ;
#11755=CARTESIAN_POINT ( 'NONE',  ( 107.0000000000000000, 110.0000000000000000, -53.49999999453763877 ) ) ;
#11787=EDGE_CURVE ( 'NONE', #23665, #7323, #17842, .T. ) ;
#11792=CARTESIAN_POINT ( 'NONE',  ( 92.99999999999998579, 110.0000000000000000, -47.00000000000001421 ) ) ;
#11796=CARTESIAN_POINT ( 'NONE',  ( 93.46109445667489979, 114.7507929638356785, -52.07499999726881867 ) ) ;
#11806=CARTESIAN_POINT ( 'NONE',  ( 97.50236033167490746, 117.6869444889999841, -46.02499999726882152 ) ) ;
#11831=CARTESIAN_POINT ( 'NONE',  ( 97.50236033167490746, 102.3130555110000159, -53.22499999726882436 ) ) ;
#11842=VECTOR ( 'NONE', #1689, 1000.000000000000000 ) ;
#11865=CARTESIAN_POINT ( 'NONE',  ( 108.0825317500000011, 110.0000000000000000, -50.87499999726882294 ) ) ;
#11884=CARTESIAN_POINT ( 'NONE',  ( 92.45873412499997812, 110.0000000000000000, -45.31249999863441502 ) ) ;
#11897=ORIENTED_EDGE ( 'NONE', *, *, #8245, .T. ) ;
#11912=CARTESIAN_POINT ( 'NONE',  ( 93.46109445667489979, 105.2492070361643215, -51.67499999726882010 ) ) ;
#11937=CARTESIAN_POINT ( 'NONE',  ( 95.00472066334982912, 116.8754121666685393, -54.17499999726881299 ) ) ;
#11946=CARTESIAN_POINT ( 'NONE',  ( 93.46109445667489979, 114.7507929638356785, -45.82499999726881867 ) ) ;
#11972=CARTESIAN_POINT ( 'NONE',  ( 104.9952793366501567, 116.8754121666685393, -54.32499999726881867 ) ) ;
#12005=CARTESIAN_POINT ( 'NONE',  ( 108.0825317500000011, 110.0000000000000000, -48.87499999726882294 ) ) ;
#12033=CARTESIAN_POINT ( 'NONE',  ( 99.99999999999998579, 110.0000000000000000, -145.0000000000000284 ) ) ;
#12046=CARTESIAN_POINT ( 'NONE',  ( 106.5389055433250860, 114.7507929638356785, -50.67499999726882010 ) ) ;
#12072=CARTESIAN_POINT ( 'NONE',  ( 93.46109445667489979, 114.7507929638356785, -54.07499999726881867 ) ) ;
#12081=CARTESIAN_POINT ( 'NONE',  ( 106.5389055433250860, 114.7507929638356785, -48.42499999726882010 ) ) ;
#12127=DIRECTION ( 'NONE',  ( 5.782411586589358625E-17, -0.000000000000000000, 1.000000000000000000 ) ) ;
#12179=ADVANCED_FACE ( 'NONE', ( #19431 ), #21577, .T. ) ;
#12184=CARTESIAN_POINT ( 'NONE',  ( 91.91746824999997045, 107.3738262389971680, -51.77499999726882152 ) ) ;
#12194=VERTEX_POINT ( 'NONE', #12983 ) ;
#12207=CARTESIAN_POINT ( 'NONE',  ( 104.3262379212492448, 115.9545556584642867, -53.19999999453762740 ) ) ;
#12216=CARTESIAN_POINT ( 'NONE',  ( 93.46109445667489979, 105.2492070361643215, -55.42499999726882720 ) ) ;
#12248=VERTEX_POINT ( 'NONE', #194 ) ;
#12258=CARTESIAN_POINT ( 'NONE',  ( 105.6631189606246153, 114.1144967660473242, -53.80000000000001137 ) ) ;
#12267=CARTESIAN_POINT ( 'NONE',  ( 99.99999999999997158, 102.6397644303321215, -50.50000000000000000 ) ) ;
#12310=CARTESIAN_POINT ( 'NONE',  ( 107.0000000000000000, 110.0000000000000000, -145.0000000000000284 ) ) ;
#12312=FACE_OUTER_BOUND ( 'NONE', #24253, .T. ) ;
#12313=CARTESIAN_POINT ( 'NONE',  ( 95.00472066334982912, 116.8754121666685393, -45.92499999726882720 ) ) ;
#12322=VECTOR ( 'NONE', #5674, 1000.000000000000000 ) ;
#12353=CARTESIAN_POINT ( 'NONE',  ( 93.00000000000000000, 112.2744378736303332, -54.59999999453764019 ) ) ;
#12356=CARTESIAN_POINT ( 'NONE',  ( 97.83688103937537051, 103.3426043859339103, -52.09999999453764019 ) ) ;
#12361=CARTESIAN_POINT ( 'NONE',  ( 95.00472066334982912, 116.8754121666685393, -51.92499999726881299 ) ) ;
#12417=PRESENTATION_STYLE_ASSIGNMENT (( #27417 ) ) ;
#12418=CARTESIAN_POINT ( 'NONE',  ( 106.9999999999999858, 107.7255621263696810, -53.59999999453763309 ) ) ;
#12421=CARTESIAN_POINT ( 'NONE',  ( 93.46109445667489979, 114.7507929638356785, -54.07499999726881867 ) ) ;
#12432=CARTESIAN_POINT ( 'NONE',  ( 102.1631189606246153, 116.6573956140660897, -47.09999999453764019 ) ) ;
#12444=CARTESIAN_POINT ( 'NONE',  ( 91.91746824999997045, 112.6261737610028320, -45.72499999726882436 ) ) ;
#12475=DIRECTION ( 'NONE',  ( -5.782411586589357392E-17, 0.000000000000000000, -1.000000000000000000 ) ) ;
#12481=DIRECTION ( 'NONE',  ( 1.000000000000000000, 0.000000000000000000, 0.000000000000000000 ) ) ;
#12482=CARTESIAN_POINT ( 'NONE',  ( 95.67376207875069838, 104.0454443415356991, -52.19999999453764872 ) ) ;
#12492=CARTESIAN_POINT ( 'NONE',  ( 97.50236033167490746, 102.3130555110000159, -51.22499999726882436 ) ) ;
#12524=( BOUNDED_CURVE ( )  B_SPLINE_CURVE ( 2, ( #27082, #20378, #20231, #18235, #714, #18085, #9536, #26944, #5270, #13935, #14910 ),
 .UNSPECIFIED., .F., .F. ) 
 B_SPLINE_CURVE_WITH_KNOTS ( ( 3, 2, 2, 2, 2, 3 ),
 ( 0.2000000000000001776, 0.2200000000000001676, 0.2400000000000001854, 0.2600000000000002309, 0.2800000000000002487, 0.3000000000000002109 ),
 .UNSPECIFIED. ) 
 CURVE ( )  GEOMETRIC_REPRESENTATION_ITEM ( )  RATIONAL_B_SPLINE_CURVE ( ( 0.9999999999999995559, 0.9510565162951539753, 1.000000000000000000, 0.9510565162951535312, 1.000000000000000000, 0.9510565162951535312, 1.000000000000000000, 0.9510565162951535312, 1.000000000000000000, 0.9510565162951529761, 1.000000000000000444 ) ) 
 REPRESENTATION_ITEM ( '' )  );
#12532=CARTESIAN_POINT ( 'NONE',  ( 95.67376207875072680, 115.9545556584642867, -53.30000000000000426 ) ) ;
#12552=CARTESIAN_POINT ( 'NONE',  ( 107.0000000000000000, 110.0000000000000000, -53.49999999453763877 ) ) ;
#12555=CARTESIAN_POINT ( 'NONE',  ( 95.00472066334982912, 116.8754121666685393, -54.17499999726881299 ) ) ;
#12560=DIRECTION ( 'NONE',  ( 0.000000000000000000, 0.000000000000000000, -1.000000000000000000 ) ) ;
#12587=EDGE_CURVE ( 'NONE', #8895, #15376, #14822, .T. ) ;
#12626=CARTESIAN_POINT ( 'NONE',  ( 94.33688103937535629, 105.8855032339526758, -50.29999999453763593 ) ) ;
#12634=CARTESIAN_POINT ( 'NONE',  ( 91.91746824999997045, 112.6261737610028320, -53.72499999726881725 ) ) ;
#12637=VECTOR ( 'NONE', #4095, 1000.000000000000000 ) ;
#12670=CARTESIAN_POINT ( 'NONE',  ( 102.1631189606246295, 103.3426043859339103, -46.40000000000001279 ) ) ;
#12694=CARTESIAN_POINT ( 'NONE',  ( 91.91746824999997045, 112.6261737610028320, -45.72499999726882436 ) ) ;
#12697=ORIENTED_EDGE ( 'NONE', *, *, #1829, .F. ) ;
#12706=AXIS2_PLACEMENT_3D ( 'NONE', #5268, #15800, #22661 ) ;
#12730=CARTESIAN_POINT ( 'NONE',  ( 91.91746824999998466, 110.0000000000000000, -47.62499999726882294 ) ) ;
#12767=CARTESIAN_POINT ( 'NONE',  ( 99.99999999999997158, 117.3602355696678501, -48.99999999453763877 ) ) ;
#12777=CARTESIAN_POINT ( 'NONE',  ( 108.0825317499999869, 107.3738262389971538, -52.72499999726881015 ) ) ;
#12788=CARTESIAN_POINT ( 'NONE',  ( 94.33688103937535629, 105.8855032339526758, -48.80000000000001137 ) ) ;
#12805=DIRECTION ( 'NONE',  ( 0.000000000000000000, 1.000000000000000000, 0.000000000000000000 ) ) ;
#12807=ORIENTED_EDGE ( 'NONE', *, *, #25863, .T. ) ;
#12832=CARTESIAN_POINT ( 'NONE',  ( 108.0825317499999869, 107.3738262389971538, -48.97499999726881015 ) ) ;
#12841=CARTESIAN_POINT ( 'NONE',  ( 94.33688103937535629, 105.8855032339526758, -54.80000000000001847 ) ) ;
#12847=( BOUNDED_CURVE ( )  B_SPLINE_CURVE ( 2, ( #16357, #14206, #22927, #1548, #23203, #8215, #14486, #10623, #3678, #3953, #4226 ),
 .UNSPECIFIED., .F., .T. ) 
 B_SPLINE_CURVE_WITH_KNOTS ( ( 3, 2, 2, 2, 2, 3 ),
 ( 0.3000000000000002109, 0.3200000000000001177, 0.3400000000000000244, 0.3599999999999998757, 0.3799999999999997824, 0.3999999999999996891 ),
 .UNSPECIFIED. ) 
 CURVE ( )  GEOMETRIC_REPRESENTATION_ITEM ( )  RATIONAL_B_SPLINE_CURVE ( ( 0.9999999999999994449, 0.9510565162951540863, 1.000000000000000000, 0.9510565162951535312, 1.000000000000000000, 0.9510565162951535312, 1.000000000000000000, 0.9510565162951535312, 1.000000000000000000, 0.9510565162951543083, 0.9999999999999992228 ) ) 
 REPRESENTATION_ITEM ( '' )  );
#12862=CARTESIAN_POINT ( 'NONE',  ( 95.00472066334982912, 103.1245878333314323, -47.32499999726881157 ) ) ;
#12896=DIRECTION ( 'NONE',  ( 5.782411586589358625E-17, -0.000000000000000000, 1.000000000000000000 ) ) ;
#12897=CARTESIAN_POINT ( 'NONE',  ( 107.0000000000000000, 112.2744378736303332, -55.39999999453763735 ) ) ;
#12900=CARTESIAN_POINT ( 'NONE',  ( 92.99999999999998579, 110.0000000000000000, -56.49999999453763877 ) ) ;
#12914=CARTESIAN_POINT ( 'NONE',  ( 94.99999999999998579, 110.0000000000000000, -145.0000000000000284 ) ) ;
#12927=DIRECTION ( 'NONE',  ( 5.782411586589358625E-17, -0.000000000000000000, 1.000000000000000000 ) ) ;
#12931=CARTESIAN_POINT ( 'NONE',  ( 107.0000000000000000, 110.0000000000000000, -53.49999999453763877 ) ) ;
#12937=CARTESIAN_POINT ( 'NONE',  ( 105.6631189606246295, 105.8855032339526758, -48.20000000000001705 ) ) ;
#12953=VECTOR ( 'NONE', #14306, 999.9999999999998863 ) ;
#12968=CARTESIAN_POINT ( 'NONE',  ( 99.99999999999997158, 101.5015231886685854, -47.37499999726882294 ) ) ;
#12976=CARTESIAN_POINT ( 'NONE',  ( 107.0000000000000000, 107.7255621263696668, -54.10000000000000853 ) ) ;
#12981=CARTESIAN_POINT ( 'NONE',  ( 92.99999999999998579, 110.0000000000000000, -56.49999999453763877 ) ) ;
#12983=CARTESIAN_POINT ( 'NONE',  ( 107.0000000000000000, 110.0000000000000000, -55.49999999453763877 ) ) ;
#12999=CARTESIAN_POINT ( 'NONE',  ( 102.4976396683250783, 102.3130555110000159, -51.02499999726882152 ) ) ;
#13036=CARTESIAN_POINT ( 'NONE',  ( 104.3262379212492448, 115.9545556584642867, -55.19999999453763451 ) ) ;
#13077=ORIENTED_EDGE ( 'NONE', *, *, #22551, .T. ) ;
#13078=CARTESIAN_POINT ( 'NONE',  ( 105.6631189606246153, 114.1144967660473242, -51.80000000000001137 ) ) ;
#13103=CARTESIAN_POINT ( 'NONE',  ( 108.0825317500000011, 110.0000000000000000, -48.62499999726882294 ) ) ;
#13105=CARTESIAN_POINT ( 'NONE',  ( 91.91746824999997045, 112.6261737610028320, -47.97499999726881725 ) ) ;
#13109=ADVANCED_FACE ( 'NONE', ( #6672 ), #21240, .T. ) ;
#13122=CARTESIAN_POINT ( 'NONE',  ( 99.99999999999998579, 110.0000000000000000, -145.0000000000000284 ) ) ;
#13143=CARTESIAN_POINT ( 'NONE',  ( 104.9952793366501709, 116.8754121666685393, -52.32499999726881867 ) ) ;
#13177=CARTESIAN_POINT ( 'NONE',  ( 97.83688103937537051, 103.3426043859339103, -56.09999999453764730 ) ) ;
#13181=CARTESIAN_POINT ( 'NONE',  ( 105.6631189606246295, 105.8855032339526758, -55.69999999453764161 ) ) ;
#13222=CARTESIAN_POINT ( 'NONE',  ( 93.00000000000000000, 112.2744378736303332, -47.10000000000001563 ) ) ;
#13246=CARTESIAN_POINT ( 'NONE',  ( 95.00472066334981491, 116.8754121666685393, -47.92499999726882720 ) ) ;
#13248=CARTESIAN_POINT ( 'NONE',  ( 99.99999999999997158, 101.5015231886685854, -49.37499999726882294 ) ) ;
#13267=EDGE_CURVE ( 'NONE', #21009, #2581, #4033, .T. ) ;
#13283=CARTESIAN_POINT ( 'NONE',  ( 108.0825317500000011, 110.0000000000000000, -54.62499999726882294 ) ) ;
#13312=CARTESIAN_POINT ( 'NONE',  ( 92.99999999999998579, 110.0000000000000000, -49.00000000000001421 ) ) ;
#13323=DIRECTION ( 'NONE',  ( 5.782411586589358625E-17, -0.000000000000000000, 1.000000000000000000 ) ) ;
#13324=CARTESIAN_POINT ( 'NONE',  ( 92.99999999999998579, 110.0000000000000000, -54.49999999453763877 ) ) ;
#13339=CARTESIAN_POINT ( 'NONE',  ( 99.99999999999997158, 118.4984768113314146, -46.37499999726881583 ) ) ;
#13367=CARTESIAN_POINT ( 'NONE',  ( 104.3262379212492448, 115.9545556584642867, -47.70000000000001705 ) ) ;
#13392=CARTESIAN_POINT ( 'NONE',  ( 104.9952793366501567, 103.1245878333314465, -46.92499999726882720 ) ) ;
#13394=CARTESIAN_POINT ( 'NONE',  ( 108.0825317499999869, 107.3738262389971538, -52.97499999726881015 ) ) ;
#13429=CARTESIAN_POINT ( 'NONE',  ( 108.0825317499999869, 107.3738262389971538, -52.72499999726881015 ) ) ;
#13430=ORIENTED_EDGE ( 'NONE', *, *, #118, .F. ) ;
#13482=CARTESIAN_POINT ( 'NONE',  ( 102.4976396683250783, 102.3130555110000159, -49.27499999726882152 ) ) ;
#13494=CARTESIAN_POINT ( 'NONE',  ( 107.0000000000000000, 112.2744378736303190, -45.90000000000000568 ) ) ;
#13509=ADVANCED_FACE ( 'NONE', ( #16913 ), #6095, .T. ) ;
#13516=EDGE_CURVE ( 'NONE', #20267, #10849, #14627, .T. ) ;
#13517=CARTESIAN_POINT ( 'NONE',  ( 104.3262379212492448, 104.0454443415356991, -50.30000000000001137 ) ) ;
#13542=CARTESIAN_POINT ( 'NONE',  ( 102.4976396683250783, 117.6869444889999841, -50.22499999726882436 ) ) ;
#13544=CARTESIAN_POINT ( 'NONE',  ( 93.46109445667489979, 105.2492070361643215, -55.67499999726882720 ) ) ;
#13551=CARTESIAN_POINT ( 'NONE',  ( 95.67376207875072680, 115.9545556584642867, -48.79999999453764303 ) ) ;
#13576=CARTESIAN_POINT ( 'NONE',  ( 91.91746824999998466, 110.0000000000000000, -49.87499999726882294 ) ) ;
#13593=CARTESIAN_POINT ( 'NONE',  ( 92.99999999999998579, 110.0000000000000000, -46.49999999453763877 ) ) ;
#13610=CARTESIAN_POINT ( 'NONE',  ( 94.33688103937534208, 114.1144967660473242, -52.69999999453764161 ) ) ;
#13661=CARTESIAN_POINT ( 'NONE',  ( 97.83688103937535629, 116.6573956140660897, -53.40000000000001990 ) ) ;
#13685=CARTESIAN_POINT ( 'NONE',  ( 99.99999999999997158, 101.5015231886685712, -53.12499999726883004 ) ) ;
#13713=EDGE_CURVE ( 'NONE', #16704, #7323, #7777, .T. ) ;
#13720=CARTESIAN_POINT ( 'NONE',  ( 108.0825317499999869, 112.6261737610028320, -48.77499999726882152 ) ) ;
#13765=CARTESIAN_POINT ( 'NONE',  ( 104.9952793366501567, 103.1245878333314465, -55.17499999726882720 ) ) ;
#13769=CARTESIAN_POINT ( 'NONE',  ( 104.3262379212492448, 104.0454443415356991, -52.30000000000001137 ) ) ;
#13797=CARTESIAN_POINT ( 'NONE',  ( 106.5389055433250860, 105.2492070361643215, -48.82499999726882578 ) ) ;
#13815=CARTESIAN_POINT ( 'NONE',  ( 99.99999999999998579, 110.0000000000000000, -145.0000000000000284 ) ) ;
#13860=CARTESIAN_POINT ( 'NONE',  ( 106.5389055433250860, 105.2492070361643215, -49.07499999726882578 ) ) ;
#13883=ORIENTED_EDGE ( 'NONE', *, *, #9595, .F. ) ;
#13908=CARTESIAN_POINT ( 'NONE',  ( 93.46109445667489979, 114.7507929638356785, -54.07499999726881867 ) ) ;
#13935=CARTESIAN_POINT ( 'NONE',  ( 107.0000000000000000, 112.2744378736303190, -47.90000000000001990 ) ) ;
#13940=CARTESIAN_POINT ( 'NONE',  ( 99.99999999999997158, 117.3602355696678501, -53.50000000000001421 ) ) ;
#13966=CARTESIAN_POINT ( 'NONE',  ( 99.99999999999997158, 118.4984768113314146, -54.12499999726881583 ) ) ;
#14005=CARTESIAN_POINT ( 'NONE',  ( 91.91746824999997045, 107.3738262389971538, -49.77499999726881441 ) ) ;
#14044=CARTESIAN_POINT ( 'NONE',  ( 92.99999999999998579, 110.0000000000000000, -51.00000000000000711 ) ) ;
#14056=CARTESIAN_POINT ( 'NONE',  ( 91.91746824999997045, 107.3738262389971680, -53.77499999726882862 ) ) ;
#14062=( GEOMETRIC_REPRESENTATION_CONTEXT ( 3 ) GLOBAL_UNCERTAINTY_ASSIGNED_CONTEXT ( ( #21825 ) ) GLOBAL_UNIT_ASSIGNED_CONTEXT ( ( #8294, #14832, #10138 ) ) REPRESENTATION_CONTEXT ( 'NONE', 'WORKASPACE' ) );
#14080=CARTESIAN_POINT ( 'NONE',  ( 107.0000000000000000, 110.0000000000000000, -47.49999999453763877 ) ) ;
#14090=CARTESIAN_POINT ( 'NONE',  ( 108.0825317499999869, 112.6261737610028320, -46.52499999726882152 ) ) ;
#14112=CARTESIAN_POINT ( 'NONE',  ( 93.46109445667489979, 105.2492070361643215, -55.42499999726882720 ) ) ;
#14134=ORIENTED_EDGE ( 'NONE', *, *, #6697, .F. ) ;
#14148=CARTESIAN_POINT ( 'NONE',  ( 106.5389055433250860, 105.2492070361643215, -47.07499999726882578 ) ) ;
#14152=ORIENTED_EDGE ( 'NONE', *, *, #1829, .T. ) ;
#14165=CARTESIAN_POINT ( 'NONE',  ( 99.99999999999997158, 117.3602355696678643, -46.99999999453763877 ) ) ;
#14167=ORIENTED_EDGE ( 'NONE', *, *, #24502, .T. ) ;
#14195=CARTESIAN_POINT ( 'NONE',  ( 102.4976396683250783, 102.3130555110000159, -51.27499999726882152 ) ) ;
#14206=CARTESIAN_POINT ( 'NONE',  ( 107.0000000000000142, 107.7255621263696668, -49.59999999453765440 ) ) ;
#14218=CARTESIAN_POINT ( 'NONE',  ( 97.83688103937537051, 103.3426043859339103, -46.60000000000000853 ) ) ;
#14221=CARTESIAN_POINT ( 'NONE',  ( 91.91746824999998466, 110.0000000000000000, -51.87499999726882294 ) ) ;
#14228=CARTESIAN_POINT ( 'NONE',  ( 102.1631189606246153, 116.6573956140660897, -53.60000000000000853 ) ) ;
#14253=CARTESIAN_POINT ( 'NONE',  ( 91.91746824999997045, 107.3738262389971680, -53.52499999726882862 ) ) ;
#14270=AXIS2_PLACEMENT_3D ( 'NONE', #15310, #6079, #4219 ) ;
#14274=CARTESIAN_POINT ( 'NONE',  ( 95.67376207875072680, 104.0454443415356991, -50.70000000000000284 ) ) ;
#14283=EDGE_CURVE ( 'NONE', #9015, #10849, #24588, .T. ) ;
#14292=CARTESIAN_POINT ( 'NONE',  ( 97.83688103937535629, 116.6573956140660897, -45.40000000000001279 ) ) ;
#14302=CARTESIAN_POINT ( 'NONE',  ( 92.99999999999998579, 112.2744378736303190, -46.59999999453763309 ) ) ;
#14306=DIRECTION ( 'NONE',  ( -0.8660254037844418162, 0.000000000000000000, -0.4999999999999947264 ) ) ;
#14309=CARTESIAN_POINT ( 'NONE',  ( 99.99999999999998579, 110.0000000000000000, -45.00000000000000711 ) ) ;
#14331=CARTESIAN_POINT ( 'NONE',  ( 99.99999999999997158, 118.4984768113314146, -54.37499999726881583 ) ) ;
#14358=CARTESIAN_POINT ( 'NONE',  ( 99.99999999999997158, 102.6397644303321215, -47.99999999453763877 ) ) ;
#14368=CARTESIAN_POINT ( 'NONE',  ( 102.4976396683250783, 102.3130555110000159, -55.02499999726882152 ) ) ;
#14385=SHAPE_DEFINITION_REPRESENTATION ( #8744, #14947 ) ;
#14391=AXIS2_PLACEMENT_3D ( 'NONE', #81, #23598, #16894 ) ;
#14401=VECTOR ( 'NONE', #15675, 1000.000000000000000 ) ;
#14428=CARTESIAN_POINT ( 'NONE',  ( 95.00472066334982912, 103.1245878333314323, -53.57499999726881157 ) ) ;
#14440=CLOSED_SHELL ( 'NONE', ( #19809, #8129, #15389, #1600, #2032, #13509, #16799, #26605, #13109, #9984, #11184, #12179, #22755, #10536, #23450, #17122, #16804, #3928, #3055, #4118, #25810 ) ) ;
#14474=EDGE_CURVE ( 'NONE', #18889, #2926, #8551, .T. ) ;
#14486=CARTESIAN_POINT ( 'NONE',  ( 97.83688103937537051, 103.3426043859339103, -50.09999999453764019 ) ) ;
#14494=CARTESIAN_POINT ( 'NONE',  ( 94.33688103937535629, 105.8855032339526758, -46.80000000000001847 ) ) ;
#14496=FACE_OUTER_BOUND ( 'NONE', #17985, .T. ) ;
#14497=CARTESIAN_POINT ( 'NONE',  ( 99.99999999999997158, 102.6397644303321215, -51.99999999453763877 ) ) ;
#14505=VECTOR ( 'NONE', #16933, 1000.000000000000000 ) ;
#14506=CARTESIAN_POINT ( 'NONE',  ( 99.99999999999997158, 101.5015231886685854, -53.12499999726883004 ) ) ;
#14535=ORIENTED_EDGE ( 'NONE', *, *, #10885, .T. ) ;
#14570=CARTESIAN_POINT ( 'NONE',  ( 108.0825317499999869, 112.6261737610028320, -54.77499999726881441 ) ) ;
#14582=CARTESIAN_POINT ( 'NONE',  ( 107.0000000000000000, 112.2744378736303190, -47.39999999453763735 ) ) ;
#14595=CARTESIAN_POINT ( 'NONE',  ( 91.91746824999998466, 110.0000000000000000, -49.62499999726882294 ) ) ;
#14596=VERTEX_POINT ( 'NONE', #16958 ) ;
#14617=CARTESIAN_POINT ( 'NONE',  ( 105.0000000000000000, 110.0000000000000000, -45.00000000000000711 ) ) ;
#14627=LINE ( 'NONE', #8362, #11842 ) ;
#14630=CARTESIAN_POINT ( 'NONE',  ( 93.00000000000000000, 112.2744378736303332, -52.59999999453764019 ) ) ;
#14639=CARTESIAN_POINT ( 'NONE',  ( 99.99999999999997158, 101.5015231886685854, -55.12499999726880873 ) ) ;
#14676=CARTESIAN_POINT ( 'NONE',  ( 99.99999999999997158, 117.3602355696678643, -53.50000000000001421 ) ) ;
#14697=CARTESIAN_POINT ( 'NONE',  ( 99.99999999999997158, 102.6397644303321215, -53.99999999453763877 ) ) ;
#14721=( NAMED_UNIT ( * ) PLANE_ANGLE_UNIT ( ) SI_UNIT ( $, .RADIAN. ) );
#14729=PLANE ( 'NONE',  #15388 ) ;
#14730=CARTESIAN_POINT ( 'NONE',  ( 108.0825317499999869, 107.3738262389971538, -46.72499999726881015 ) ) ;
#14766=CARTESIAN_POINT ( 'NONE',  ( 107.0000000000000000, 107.7255621263696668, -51.59999999453763309 ) ) ;
#14789=CARTESIAN_POINT ( 'NONE',  ( 105.0000000000000000, 110.0000000000000000, -145.0000000000000284 ) ) ;
#14803=CARTESIAN_POINT ( 'NONE',  ( 104.3262379212492448, 115.9545556584642867, -45.70000000000001705 ) ) ;
#14822=LINE ( 'NONE', #25672, #21427 ) ;
#14830=CARTESIAN_POINT ( 'NONE',  ( 108.0825317500000011, 110.0000000000000000, -48.87499999726882294 ) ) ;
#14832=( NAMED_UNIT ( * ) PLANE_ANGLE_UNIT ( ) SI_UNIT ( $, .RADIAN. ) );
#14833=AXIS2_PLACEMENT_3D ( 'NONE', #24414, #11285, #17181 ) ;
#14837=CARTESIAN_POINT ( 'NONE',  ( 97.50236033167490746, 102.3130555110000159, -55.47499999726881725 ) ) ;
#14901=CARTESIAN_POINT ( 'NONE',  ( 99.99999999999998579, 110.0000000000000000, -145.0000000000000284 ) ) ;
#14905=CARTESIAN_POINT ( 'NONE',  ( 95.67376207875069838, 104.0454443415356991, -50.19999999453764161 ) ) ;
#14910=CARTESIAN_POINT ( 'NONE',  ( 107.0000000000000000, 110.0000000000000000, -48.00000000000001421 ) ) ;
#14914=CARTESIAN_POINT ( 'NONE',  ( 93.46109445667489979, 114.7507929638356785, -51.82499999726881867 ) ) ;
#14919=( GEOMETRIC_REPRESENTATION_CONTEXT ( 3 ) GLOBAL_UNCERTAINTY_ASSIGNED_CONTEXT ( ( #25165 ) ) GLOBAL_UNIT_ASSIGNED_CONTEXT ( ( #10302, #14721, #19009 ) ) REPRESENTATION_CONTEXT ( 'NONE', 'WORKASPACE' ) );
#14928=CARTESIAN_POINT ( 'NONE',  ( 104.3262379212492448, 104.0454443415356991, -48.30000000000001137 ) ) ;
#14940=VECTOR ( 'NONE', #13323, 1000.000000000000000 ) ;
#14947=SHAPE_REPRESENTATION ( 'main air inlet', ( #26844 ), #10431 ) ;
#14975=CARTESIAN_POINT ( 'NONE',  ( 104.9952793366501709, 116.8754121666685393, -50.57499999726882578 ) ) ;
#14978=CARTESIAN_POINT ( 'NONE',  ( 105.6631189606246295, 105.8855032339526758, -53.69999999453763451 ) ) ;
#14988=ORIENTED_EDGE ( 'NONE', *, *, #22584, .F. ) ;
#14996=ORIENTED_EDGE ( 'NONE', *, *, #3729, .T. ) ;
#15007=CARTESIAN_POINT ( 'NONE',  ( 106.5389055433250860, 114.7507929638356785, -48.42499999726882010 ) ) ;
#15042=CARTESIAN_POINT ( 'NONE',  ( 99.99999999999998579, 110.0000000000000000, -145.0000000000000284 ) ) ;
#15044=CARTESIAN_POINT ( 'NONE',  ( 105.6631189606246295, 105.8855032339526758, -49.69999999453764161 ) ) ;
#15059=FACE_OUTER_BOUND ( 'NONE', #20455, .T. ) ;
#15082=CARTESIAN_POINT ( 'NONE',  ( 102.1631189606246153, 116.6573956140660897, -47.60000000000000853 ) ) ;
#15110=CARTESIAN_POINT ( 'NONE',  ( 108.0825317499999869, 107.3738262389971538, -46.97499999726881015 ) ) ;
#15119=FACE_OUTER_BOUND ( 'NONE', #24993, .T. ) ;
#15146=CARTESIAN_POINT ( 'NONE',  ( 99.99999999999997158, 118.4984768113314004, -54.12499999726881583 ) ) ;
#15194=CARTESIAN_POINT ( 'NONE',  ( 108.0825317499999869, 107.3738262389971680, -48.97499999726881725 ) ) ;
#15226=CARTESIAN_POINT ( 'NONE',  ( 104.3262379212492448, 115.9545556584642867, -49.70000000000001705 ) ) ;
#15252=CARTESIAN_POINT ( 'NONE',  ( 97.50236033167490746, 117.6869444889999841, -48.02499999726882152 ) ) ;
#15255=CARTESIAN_POINT ( 'NONE',  ( 91.91746824999998466, 110.0000000000000000, -49.87499999726882294 ) ) ;
#15263=CARTESIAN_POINT ( 'NONE',  ( 91.91746824999998466, 110.0000000000000000, -45.74999999726882294 ) ) ;
#15269=DIRECTION ( 'NONE',  ( 5.782411586589358625E-17, -0.000000000000000000, 1.000000000000000000 ) ) ;
#15292=CARTESIAN_POINT ( 'NONE',  ( 93.46109445667489979, 114.7507929638356785, -46.07499999726881867 ) ) ;
#15310=CARTESIAN_POINT ( 'NONE',  ( 99.99999999999998579, 110.0000000000000000, -45.00000000000000711 ) ) ;
#15328=CARTESIAN_POINT ( 'NONE',  ( 94.33688103937534208, 114.1144967660473242, -49.20000000000001705 ) ) ;
#15340=CARTESIAN_POINT ( 'NONE',  ( 99.99999999999997158, 101.5015231886685712, -47.37499999726882294 ) ) ;
#15369=CARTESIAN_POINT ( 'NONE',  ( 97.83688103937537051, 103.3426043859339103, -50.60000000000001563 ) ) ;
#15376=VERTEX_POINT ( 'NONE', #12981 ) ;
#15388=AXIS2_PLACEMENT_3D ( 'NONE', #12033, #21169, #16881 ) ;
#15389=ADVANCED_FACE ( 'NONE', ( #23708 ), #19703, .T. ) ;
#15397=CARTESIAN_POINT ( 'NONE',  ( 106.5389055433250860, 105.2492070361643215, -48.82499999726882578 ) ) ;
#15399=CARTESIAN_POINT ( 'NONE',  ( 97.50236033167490746, 102.3130555110000159, -51.47499999726882436 ) ) ;
#15403=CARTESIAN_POINT ( 'NONE',  ( 94.99999999999998579, 110.0000000000000000, -145.0000000000000284 ) ) ;
#15415=EDGE_CURVE ( 'NONE', #9571, #499, #7214, .T. ) ;
#15435=CARTESIAN_POINT ( 'NONE',  ( 95.00472066334982912, 116.8754121666685393, -53.92499999726881299 ) ) ;
#15470=CARTESIAN_POINT ( 'NONE',  ( 107.0000000000000000, 110.0000000000000000, -55.49999999453763877 ) ) ;
#15484=CARTESIAN_POINT ( 'NONE',  ( 91.91746824999997045, 112.6261737610028320, -47.97499999726881725 ) ) ;
#15496=CARTESIAN_POINT ( 'NONE',  ( 92.99999999999998579, 110.0000000000000000, -45.00000000000001421 ) ) ;
#15518=CARTESIAN_POINT ( 'NONE',  ( 107.0000000000000000, 112.2744378736303332, -49.90000000000000568 ) ) ;
#15541=CARTESIAN_POINT ( 'NONE',  ( 99.99999999999997158, 118.4984768113314146, -48.12499999726881583 ) ) ;
#15543=CARTESIAN_POINT ( 'NONE',  ( 104.9952793366501709, 103.1245878333314323, -53.17499999726882010 ) ) ;
#15557=CARTESIAN_POINT ( 'NONE',  ( 99.99999999999998579, 110.0000000000000000, -45.00000000000000711 ) ) ;
#15579=CARTESIAN_POINT ( 'NONE',  ( 104.9952793366501709, 116.8754121666685393, -50.32499999726882578 ) ) ;
#15618=CARTESIAN_POINT ( 'NONE',  ( 107.0000000000000000, 107.7255621263696668, -55.59999999453763309 ) ) ;
#15620=ORIENTED_EDGE ( 'NONE', *, *, #1675, .T. ) ;
#15635=CARTESIAN_POINT ( 'NONE',  ( 91.91746824999997045, 107.3738262389971680, -49.77499999726881441 ) ) ;
#15643=CARTESIAN_POINT ( 'NONE',  ( 105.6631189606246295, 105.8855032339526758, -47.69999999453764161 ) ) ;
#15665=CARTESIAN_POINT ( 'NONE',  ( 107.0000000000000000, 110.0000000000000000, -50.00000000000000711 ) ) ;
#15675=DIRECTION ( 'NONE',  ( 5.782411586589358625E-17, -0.000000000000000000, 1.000000000000000000 ) ) ;
#15688=CARTESIAN_POINT ( 'NONE',  ( 95.00472066334981491, 116.8754121666685393, -49.92499999726880588 ) ) ;
#15690=CARTESIAN_POINT ( 'NONE',  ( 105.6631189606246153, 114.1144967660473242, -47.29999999453764303 ) ) ;
#15700=ORIENTED_EDGE ( 'NONE', *, *, #16294, .F. ) ;
#15724=CARTESIAN_POINT ( 'NONE',  ( 91.91746824999997045, 112.6261737610028320, -45.97499999726882436 ) ) ;
#15729=ORIENTED_EDGE ( 'NONE', *, *, #14283, .T. ) ;
#15759=CARTESIAN_POINT ( 'NONE',  ( 93.00000000000001421, 112.2744378736303617, -49.10000000000000142 ) ) ;
#15800=DIRECTION ( 'NONE',  ( 5.782411586589358625E-17, -0.000000000000000000, 1.000000000000000000 ) ) ;
#15805=CARTESIAN_POINT ( 'NONE',  ( 93.46109445667489979, 105.2492070361643215, -49.42499999726882010 ) ) ;
#15829=CARTESIAN_POINT ( 'NONE',  ( 106.5389055433250860, 114.7507929638356785, -52.42499999726882010 ) ) ;
#15853=CYLINDRICAL_SURFACE ( 'NONE', #14833, 7.000000000000006217 ) ;
#15864=CARTESIAN_POINT ( 'NONE',  ( 91.91746824999998466, 110.0000000000000000, -47.87499999726882294 ) ) ;
#15887=COLOUR_RGB ( '', 0.66274510, 0.83137255, 0.94901961) ;
#15906=CARTESIAN_POINT ( 'NONE',  ( 108.0825317499999869, 112.6261737610028320, -52.77499999726883573 ) ) ;
#15919=CARTESIAN_POINT ( 'NONE',  ( 102.1631189606246153, 116.6573956140660897, -45.60000000000001563 ) ) ;
#15930=EDGE_CURVE ( 'NONE', #3337, #24121, #21372, .T. ) ;
#15942=CARTESIAN_POINT ( 'NONE',  ( 91.91746824999997045, 107.3738262389971538, -47.52499999726881441 ) ) ;
#16004=CARTESIAN_POINT ( 'NONE',  ( 95.00472066334982912, 116.8754121666685393, -52.17499999726881299 ) ) ;
#16014=DIRECTION ( 'NONE',  ( 5.782411586589358625E-17, -0.000000000000000000, 1.000000000000000000 ) ) ;
#16053=CARTESIAN_POINT ( 'NONE',  ( 91.91746824999997045, 107.3738262389971680, -55.77499999726881441 ) ) ;
#16063=DIRECTION ( 'NONE',  ( 0.8660254037844418162, -0.000000000000000000, 0.4999999999999947264 ) ) ;
#16086=CARTESIAN_POINT ( 'NONE',  ( 91.91746824999998466, 110.0000000000000000, -47.62499999726882294 ) ) ;
#16117=DIRECTION ( 'NONE',  ( -5.782411586589357392E-17, 0.000000000000000000, -1.000000000000000000 ) ) ;
#16150=CARTESIAN_POINT ( 'NONE',  ( 97.50236033167490746, 117.6869444889999841, -52.27499999726882862 ) ) ;
#16156=FACE_OUTER_BOUND ( 'NONE', #9593, .T. ) ;
#16213=( BOUNDED_CURVE ( )  B_SPLINE_CURVE ( 2, ( #26056, #11210, #15643, #21791, #4256, #19503, #22074, #265, #2123, #4539, #123 ),
 .UNSPECIFIED., .F., .F. ) 
 B_SPLINE_CURVE_WITH_KNOTS ( ( 3, 2, 2, 2, 2, 3 ),
 ( 0.1000000000000000056, 0.1200000000000000233, 0.1400000000000000688, 0.1600000000000001144, 0.1800000000000001044, 0.2000000000000001776 ),
 .UNSPECIFIED. ) 
 CURVE ( )  GEOMETRIC_REPRESENTATION_ITEM ( )  RATIONAL_B_SPLINE_CURVE ( ( 1.000000000000000000, 0.9510565162951535312, 1.000000000000000000, 0.9510565162951535312, 1.000000000000000000, 0.9510565162951535312, 1.000000000000000000, 0.9510565162951535312, 1.000000000000000000, 0.9510565162951530871, 1.000000000000000444 ) ) 
 REPRESENTATION_ITEM ( '' )  );
#16226=CARTESIAN_POINT ( 'NONE',  ( 99.99999999999997158, 117.3602355696678501, -46.99999999453764588 ) ) ;
#16229=ORIENTED_EDGE ( 'NONE', *, *, #12587, .F. ) ;
#16237=CARTESIAN_POINT ( 'NONE',  ( 102.4976396683250783, 102.3130555110000159, -49.02499999726882152 ) ) ;
#16294=EDGE_CURVE ( 'NONE', #27236, #24786, #6433, .T. ) ;
#16298=CARTESIAN_POINT ( 'NONE',  ( 91.91746824999997045, 107.3738262389971538, -47.77499999726880731 ) ) ;
#16302=CARTESIAN_POINT ( 'NONE',  ( 105.6631189606246153, 114.1144967660473242, -45.80000000000001137 ) ) ;
#16309=ORIENTED_EDGE ( 'NONE', *, *, #16663, .F. ) ;
#16341=EDGE_CURVE ( 'NONE', #19908, #14596, #16491, .T. ) ;
#16346=CARTESIAN_POINT ( 'NONE',  ( 106.5389055433250860, 105.2492070361643215, -55.07499999726882578 ) ) ;
#16357=CARTESIAN_POINT ( 'NONE',  ( 107.0000000000000000, 110.0000000000000000, -49.49999999453764588 ) ) ;
#16368=CARTESIAN_POINT ( 'NONE',  ( 91.91746824999998466, 110.0000000000000000, -55.87499999726882294 ) ) ;
#16377=CARTESIAN_POINT ( 'NONE',  ( 107.0000000000000000, 112.2744378736303332, -53.90000000000000568 ) ) ;
#16405=CARTESIAN_POINT ( 'NONE',  ( 108.0825317499999869, 107.3738262389971680, -52.72499999726881725 ) ) ;
#16435=CARTESIAN_POINT ( 'NONE',  ( 97.50236033167490746, 102.3130555110000159, -49.47499999726882436 ) ) ;
#16461=DIRECTION ( 'NONE',  ( -5.782411586589357392E-17, 0.000000000000000000, -1.000000000000000000 ) ) ;
#16464=DIRECTION ( 'NONE',  ( 5.782411586589358625E-17, -0.000000000000000000, 1.000000000000000000 ) ) ;
#16483=CARTESIAN_POINT ( 'NONE',  ( 97.50236033167490746, 117.6869444889999841, -54.27499999726882862 ) ) ;
#16491=LINE ( 'NONE', #25186, #12322 ) ;
#16512=CARTESIAN_POINT ( 'NONE',  ( 107.0000000000000000, 112.2744378736303332, -47.39999999453763735 ) ) ;
#16520=CARTESIAN_POINT ( 'NONE',  ( 93.46109445667489979, 114.7507929638356785, -53.82499999726881867 ) ) ;
#16566=LINE ( 'NONE', #9868, #1665 ) ;
#16577=CARTESIAN_POINT ( 'NONE',  ( 106.5389055433250860, 114.7507929638356785, -54.67499999726882720 ) ) ;
#16598=( LENGTH_UNIT ( ) NAMED_UNIT ( * ) SI_UNIT ( .MILLI., .METRE. ) );
#16609=CARTESIAN_POINT ( 'NONE',  ( 104.9952793366501709, 103.1245878333314323, -48.92499999726882010 ) ) ;
#16613=UNCERTAINTY_MEASURE_WITH_UNIT (LENGTH_MEASURE( 1.000000000000000082E-05 ), #16598, 'distance_accuracy_value', 'NONE');
#16649=CARTESIAN_POINT ( 'NONE',  ( 93.00000000000000000, 107.7255621263696526, -54.39999999453763024 ) ) ;
#16659=CARTESIAN_POINT ( 'NONE',  ( 102.4976396683250783, 117.6869444889999841, -52.22499999726882436 ) ) ;
#16661=AXIS2_PLACEMENT_3D ( 'NONE', #15042, #19480, #23759 ) ;
#16663=EDGE_CURVE ( 'NONE', #18889, #8895, #26077, .T. ) ;
#16704=VERTEX_POINT ( 'NONE', #10712 ) ;
#16711=AXIS2_PLACEMENT_3D ( 'NONE', #26100, #28104, #8568 ) ;
#16719=CARTESIAN_POINT ( 'NONE',  ( 104.3262379212492448, 104.0454443415356991, -53.79999999453763593 ) ) ;
#16747=CARTESIAN_POINT ( 'NONE',  ( 95.00472066334982912, 103.1245878333314323, -49.32499999726881157 ) ) ;
#16785=CARTESIAN_POINT ( 'NONE',  ( 105.6631189606246153, 114.1144967660473242, -53.29999999453764303 ) ) ;
#16793=CARTESIAN_POINT ( 'NONE',  ( 102.4976396683250783, 102.3130555110000159, -51.02499999726882152 ) ) ;
#16799=ADVANCED_FACE ( 'NONE', ( #17417 ), #3898, .T. ) ;
#16804=ADVANCED_FACE ( 'NONE', ( #15119 ), #6581, .T. ) ;
#16881=DIRECTION ( 'NONE',  ( -1.000000000000000000, 0.000000000000000000, 5.782411586589357392E-17 ) ) ;
#16894=DIRECTION ( 'NONE',  ( -1.000000000000000000, 0.000000000000000000, 0.000000000000000000 ) ) ;
#16913=FACE_OUTER_BOUND ( 'NONE', #26238, .T. ) ;
#16916=CARTESIAN_POINT ( 'NONE',  ( 95.67376207875069838, 104.0454443415356991, -54.19999999453764161 ) ) ;
#16920=( BOUNDED_CURVE ( )  B_SPLINE_CURVE ( 2, ( #28047, #6241, #13181, #21920, #28184, #17343, #25904, #22055, #21488, #1969, #12900 ),
 .UNSPECIFIED., .F., .F. ) 
 B_SPLINE_CURVE_WITH_KNOTS ( ( 3, 2, 2, 2, 2, 3 ),
 ( 0.9000000000000000222, 0.9200000000000000400, 0.9399999999999999467, 0.9599999999999999645, 0.9799999999999999822, 1.000000000000000000 ),
 .UNSPECIFIED. ) 
 CURVE ( )  GEOMETRIC_REPRESENTATION_ITEM ( )  RATIONAL_B_SPLINE_CURVE ( ( 1.000000000000000000, 0.9510565162951535312, 1.000000000000000000, 0.9510565162951535312, 1.000000000000000000, 0.9510565162951535312, 1.000000000000000000, 0.9510565162951535312, 1.000000000000000000, 0.9510565162951535312, 1.000000000000000000 ) ) 
 REPRESENTATION_ITEM ( '' )  );
#16933=DIRECTION ( 'NONE',  ( 5.782411586589358625E-17, -0.000000000000000000, 1.000000000000000000 ) ) ;
#16953=VECTOR ( 'NONE', #16063, 999.9999999999998863 ) ;
#16958=CARTESIAN_POINT ( 'NONE',  ( 91.91746824999998466, 110.0000000000000000, -55.62499999726882294 ) ) ;
#16975=CARTESIAN_POINT ( 'NONE',  ( 91.91746824999998466, 110.0000000000000000, -45.62499999726882294 ) ) ;
#16983=CARTESIAN_POINT ( 'NONE',  ( 91.91746824999998466, 110.0000000000000000, -45.87499999726882294 ) ) ;
#16987=CARTESIAN_POINT ( 'NONE',  ( 108.0825317500000011, 110.0000000000000000, -54.87499999726882294 ) ) ;
#16992=CARTESIAN_POINT ( 'NONE',  ( 99.99999999999997158, 102.6397644303321215, -54.50000000000000711 ) ) ;
#17026=( BOUNDED_SURFACE ( )  B_SPLINE_SURFACE ( 1, 2, ( 
 ( #21454, #12444, #8329, #12313, #1380, #23314, #3649, #7914, #1651, #6064, #28008, #14730, #27591, #23449, #21309, #10171, #23584, #12862, #25717, #6200, #12730, #1932, #10600, #8472, #21034, #17159, #25861, #6333, #15007, #23729, #10041, #18753, #27453, #16609, #25303, #5790, #8051, #16747, #25447, #5928, #14595, #3786, #6749, #19867, #6472, #10877, #17299, #15579, #6893, #11010, #19723, #8751, #4916, #4343, #12999, #24009, #4767, #9179, #21879, #8894, #24427, #2490, #21591, #4626, #26141, #209, #19446, #13143, #26001, #17872, #28144, #13429, #17442, #2067, #10737, #17584, #26289, #19586, #21738, #22157, #498, #4486, #11295, #15435, #22013, #15146, #8612, #24149, #2355, #26434, #13283, #24286, #11151, #23864, #2212, #2635, #69, #20018, #353, #9038, #26577 ),
 ( #7026, #15724, #15292, #17732, #6607, #7167, #11439, #3335, #1071, #22442, #1213, #5339, #14148, #9879, #18585, #27155, #7607, #24574, #22586, #16298, #15864, #3054, #928, #18011, #24999, #22867, #5055, #9740, #5478, #13720, #12005, #18448, #13860, #20729, #27291, #7747, #16435, #18155, #25132, #14005, #13576, #22300, #18301, #5196, #20159, #2775, #640, #9599, #9313, #26721, #11865, #2909, #11578, #24718, #20298, #7456, #785, #9455, #11721, #26869, #20447, #7315, #27009, #16004, #16150, #24858, #22728, #3194, #20588, #10429, #27978, #18993, #4037, #3759, #1487, #10571, #21281, #14428, #10014, #20866, #19137, #8437, #12421, #12555, #10284, #19280, #27843, #8299, #16577, #14570, #16987, #27421, #23285, #21139, #18723, #25687, #14837, #7884, #1764, #6170, #25270 ) ),
 .UNSPECIFIED., .F., .F., .T. ) 
 B_SPLINE_SURFACE_WITH_KNOTS ( ( 2, 2 ),
 ( 3, 2, 2, 2, 2, 2, 2, 2, 2, 2, 2, 2, 2, 2, 2, 2, 2, 2, 2, 2, 2, 2, 2, 2, 2, 2, 2, 2, 2, 2, 2, 2, 2, 2, 2, 2, 2, 2, 2, 2, 2, 2, 2, 2, 2, 2, 2, 2, 2, 2, 3 ),
 ( 0.000000000000000000, 1.000000000000000000 ),
 ( 0.000000000000000000, 0.02000000000000000042, 0.04000000000000000083, 0.05999999999999999778, 0.08000000000000000167, 0.1000000000000000056, 0.1199999999999999956, 0.1400000000000000133, 0.1600000000000000033, 0.1799999999999999933, 0.2000000000000000111, 0.2200000000000000011, 0.2399999999999999911, 0.2600000000000000089, 0.2800000000000000266, 0.2999999999999999889, 0.3200000000000000067, 0.3400000000000000244, 0.3599999999999999867, 0.3800000000000000044, 0.4000000000000000222, 0.4199999999999999845, 0.4400000000000000022, 0.4600000000000000200, 0.4799999999999999822, 0.5000000000000000000, 0.5200000000000000178, 0.5400000000000000355, 0.5600000000000000533, 0.5799999999999999600, 0.5999999999999999778, 0.6199999999999999956, 0.6400000000000000133, 0.6600000000000000311, 0.6800000000000000488, 0.6999999999999999556, 0.7199999999999999734, 0.7399999999999999911, 0.7600000000000000089, 0.7800000000000000266, 0.8000000000000000444, 0.8199999999999999512, 0.8399999999999999689, 0.8599999999999999867, 0.8800000000000000044, 0.9000000000000000222, 0.9200000000000000400, 0.9399999999999999467, 0.9599999999999999645, 0.9799999999999999822, 1.000000000000000000 ),
 .UNSPECIFIED. ) 
 GEOMETRIC_REPRESENTATION_ITEM ( )  RATIONAL_B_SPLINE_SURFACE ( (
 ( 1.000000000000000000, 0.9510565162951535312, 1.000000000000000000, 0.9510565162951535312, 1.000000000000000000, 0.9510565162951535312, 1.000000000000000000, 0.9510565162951535312, 1.000000000000000000, 0.9510565162951535312, 1.000000000000000000, 0.9510565162951535312, 1.000000000000000000, 0.9510565162951535312, 1.000000000000000000, 0.9510565162951535312, 1.000000000000000000, 0.9510565162951535312, 1.000000000000000000, 0.9510565162951535312, 1.000000000000000000, 0.9510565162951535312, 1.000000000000000000, 0.9510565162951535312, 1.000000000000000000, 0.9510565162951535312, 1.000000000000000000, 0.9510565162951535312, 1.000000000000000000, 0.9510565162951535312, 1.000000000000000000, 0.9510565162951535312, 1.000000000000000000, 0.9510565162951535312, 1.000000000000000000, 0.9510565162951535312, 1.000000000000000000, 0.9510565162951535312, 1.000000000000000000, 0.9510565162951535312, 1.000000000000000000, 0.9510565162951535312, 1.000000000000000000, 0.9510565162951535312, 1.000000000000000000, 0.9510565162951535312, 1.000000000000000000, 0.9510565162951535312, 1.000000000000000000, 0.9510565162951535312, 1.000000000000000000, 0.9510565162951535312, 1.000000000000000000, 0.9510565162951535312, 1.000000000000000000, 0.9510565162951535312, 1.000000000000000000, 0.9510565162951535312, 1.000000000000000000, 0.9510565162951535312, 1.000000000000000000, 0.9510565162951535312, 1.000000000000000000, 0.9510565162951535312, 1.000000000000000000, 0.9510565162951535312, 1.000000000000000000, 0.9510565162951535312, 1.000000000000000000, 0.9510565162951535312, 1.000000000000000000, 0.9510565162951535312, 1.000000000000000000, 0.9510565162951535312, 1.000000000000000000, 0.9510565162951535312, 1.000000000000000000, 0.9510565162951535312, 1.000000000000000000, 0.9510565162951535312, 1.000000000000000000, 0.9510565162951535312, 1.000000000000000000, 0.9510565162951535312, 1.000000000000000000, 0.9510565162951535312, 1.000000000000000000, 0.9510565162951535312, 1.000000000000000000, 0.9510565162951535312, 1.000000000000000000, 0.9510565162951535312, 1.000000000000000000, 0.9510565162951535312, 1.000000000000000000, 0.9510565162951535312, 1.000000000000000000, 0.9510565162951535312, 1.000000000000000000, 0.9510565162951535312, 1.000000000000000000),
 ( 1.000000000000000000, 0.9510565162951535312, 1.000000000000000000, 0.9510565162951535312, 1.000000000000000000, 0.9510565162951535312, 1.000000000000000000, 0.9510565162951535312, 1.000000000000000000, 0.9510565162951535312, 1.000000000000000000, 0.9510565162951535312, 1.000000000000000000, 0.9510565162951535312, 1.000000000000000000, 0.9510565162951535312, 1.000000000000000000, 0.9510565162951535312, 1.000000000000000000, 0.9510565162951535312, 1.000000000000000000, 0.9510565162951535312, 1.000000000000000000, 0.9510565162951535312, 1.000000000000000000, 0.9510565162951535312, 1.000000000000000000, 0.9510565162951535312, 1.000000000000000000, 0.9510565162951535312, 1.000000000000000000, 0.9510565162951535312, 1.000000000000000000, 0.9510565162951535312, 1.000000000000000000, 0.9510565162951535312, 1.000000000000000000, 0.9510565162951535312, 1.000000000000000000, 0.9510565162951535312, 1.000000000000000000, 0.9510565162951535312, 1.000000000000000000, 0.9510565162951535312, 1.000000000000000000, 0.9510565162951535312, 1.000000000000000000, 0.9510565162951535312, 1.000000000000000000, 0.9510565162951535312, 1.000000000000000000, 0.9510565162951535312, 1.000000000000000000, 0.9510565162951535312, 1.000000000000000000, 0.9510565162951535312, 1.000000000000000000, 0.9510565162951535312, 1.000000000000000000, 0.9510565162951535312, 1.000000000000000000, 0.9510565162951535312, 1.000000000000000000, 0.9510565162951535312, 1.000000000000000000, 0.9510565162951535312, 1.000000000000000000, 0.9510565162951535312, 1.000000000000000000, 0.9510565162951535312, 1.000000000000000000, 0.9510565162951535312, 1.000000000000000000, 0.9510565162951535312, 1.000000000000000000, 0.9510565162951535312, 1.000000000000000000, 0.9510565162951535312, 1.000000000000000000, 0.9510565162951535312, 1.000000000000000000, 0.9510565162951535312, 1.000000000000000000, 0.9510565162951535312, 1.000000000000000000, 0.9510565162951535312, 1.000000000000000000, 0.9510565162951535312, 1.000000000000000000, 0.9510565162951535312, 1.000000000000000000, 0.9510565162951535312, 1.000000000000000000, 0.9510565162951535312, 1.000000000000000000, 0.9510565162951535312, 1.000000000000000000, 0.9510565162951535312, 1.000000000000000000, 0.9510565162951535312, 1.000000000000000000) ) ) 
 REPRESENTATION_ITEM ( '' )  SURFACE ( )  );
#17051=CARTESIAN_POINT ( 'NONE',  ( 97.83688103937535629, 116.6573956140660897, -54.89999999453763735 ) ) ;
#17060=CARTESIAN_POINT ( 'NONE',  ( 104.9952793366501709, 103.1245878333314323, -52.92499999726882010 ) ) ;
#17118=CARTESIAN_POINT ( 'NONE',  ( 97.50236033167490746, 117.6869444889999841, -46.02499999726882152 ) ) ;
#17120=CARTESIAN_POINT ( 'NONE',  ( 93.46109445667489979, 114.7507929638356785, -46.07499999726881867 ) ) ;
#17122=ADVANCED_FACE ( 'NONE', ( #24268 ), #51, .F. ) ;
#17124=AXIS2_PLACEMENT_3D ( 'NONE', #10000, #24848, #1059 ) ;
#17133=CARTESIAN_POINT ( 'NONE',  ( 95.67376207875072680, 104.0454443415356991, -54.70000000000000995 ) ) ;
#17159=CARTESIAN_POINT ( 'NONE',  ( 99.99999999999997158, 118.4984768113314004, -48.12499999726881583 ) ) ;
#17181=DIRECTION ( 'NONE',  ( 1.000000000000000000, 0.000000000000000000, 0.000000000000000000 ) ) ;
#17194=CARTESIAN_POINT ( 'NONE',  ( 105.6631189606246295, 105.8855032339526758, -53.69999999453763451 ) ) ;
#17249=CARTESIAN_POINT ( 'NONE',  ( 92.99999999999998579, 110.0000000000000000, -52.49999999453763877 ) ) ;
#17266=CARTESIAN_POINT ( 'NONE',  ( 104.9952793366501709, 103.1245878333314323, -51.17499999726881299 ) ) ;
#17299=CARTESIAN_POINT ( 'NONE',  ( 102.4976396683250783, 117.6869444889999841, -50.22499999726882436 ) ) ;
#17339=CARTESIAN_POINT ( 'NONE',  ( 94.33688103937535629, 105.8855032339526758, -56.29999999453763593 ) ) ;
#17343=CARTESIAN_POINT ( 'NONE',  ( 99.99999999999997158, 102.6397644303321215, -55.99999999453763877 ) ) ;
#17367=CARTESIAN_POINT ( 'NONE',  ( 107.0000000000000000, 110.0000000000000000, -51.49999999453763877 ) ) ;
#17380=CARTESIAN_POINT ( 'NONE',  ( 93.00000000000000000, 107.7255621263696526, -46.90000000000001279 ) ) ;
#17383=CARTESIAN_POINT ( 'NONE',  ( 107.0000000000000000, 110.0000000000000000, -145.0000000000000284 ) ) ;
#17405=CARTESIAN_POINT ( 'NONE',  ( 108.0825317499999869, 107.3738262389971680, -48.72499999726881725 ) ) ;
#17408=CARTESIAN_POINT ( 'NONE',  ( 93.46109445667489979, 114.7507929638356785, -48.07499999726882578 ) ) ;
#17417=FACE_OUTER_BOUND ( 'NONE', #2997, .T. ) ;
#17442=CARTESIAN_POINT ( 'NONE',  ( 106.5389055433250860, 105.2492070361643215, -52.82499999726881867 ) ) ;
#17462=ORIENTED_EDGE ( 'NONE', *, *, #10203, .F. ) ;
#17475=CARTESIAN_POINT ( 'NONE',  ( 106.9999999999999716, 112.2744378736303759, -49.90000000000000568 ) ) ;
#17485=ORIENTED_EDGE ( 'NONE', *, *, #3729, .F. ) ;
#17490=CARTESIAN_POINT ( 'NONE',  ( 97.50236033167490746, 117.6869444889999841, -46.27499999726882152 ) ) ;
#17521=CARTESIAN_POINT ( 'NONE',  ( 94.33688103937535629, 105.8855032339526758, -48.80000000000001137 ) ) ;
#17547=CARTESIAN_POINT ( 'NONE',  ( 91.91746824999998466, 110.0000000000000000, -51.62499999726882294 ) ) ;
#17549=CARTESIAN_POINT ( 'NONE',  ( 108.0825317500000011, 110.0000000000000000, -50.87499999726882294 ) ) ;
#17584=CARTESIAN_POINT ( 'NONE',  ( 99.99999999999997158, 101.5015231886685854, -53.12499999726883004 ) ) ;
#17630=CARTESIAN_POINT ( 'NONE',  ( 95.00472066334981491, 103.1245878333314465, -49.57499999726881157 ) ) ;
#17661=CIRCLE ( 'NONE', #20872, 5.000000000000004441 ) ;
#17663=CARTESIAN_POINT ( 'NONE',  ( 99.99999999999997158, 102.6397644303321215, -48.50000000000000711 ) ) ;
#17668=ORIENTED_EDGE ( 'NONE', *, *, #6201, .F. ) ;
#17694=CARTESIAN_POINT ( 'NONE',  ( 99.99999999999997158, 101.5015231886685712, -51.12499999726882294 ) ) ;
#17697=CARTESIAN_POINT ( 'NONE',  ( 97.83688103937537051, 103.3426043859339103, -48.09999999453764019 ) ) ;
#17732=CARTESIAN_POINT ( 'NONE',  ( 95.00472066334982912, 116.8754121666685393, -46.17499999726882720 ) ) ;
#17767=CARTESIAN_POINT ( 'NONE',  ( 97.83688103937535629, 116.6573956140660897, -49.40000000000001279 ) ) ;
#17781=CARTESIAN_POINT ( 'NONE',  ( 106.5389055433250860, 114.7507929638356785, -46.67499999726882720 ) ) ;
#17791=CARTESIAN_POINT ( 'NONE',  ( 107.0000000000000000, 110.0000000000000000, -46.00000000000001421 ) ) ;
#17810=CARTESIAN_POINT ( 'NONE',  ( 92.99999999999998579, 110.0000000000000000, -47.00000000000001421 ) ) ;
#17833=CARTESIAN_POINT ( 'NONE',  ( 104.9952793366501567, 116.8754121666685393, -50.32499999726882578 ) ) ;
#17835=CARTESIAN_POINT ( 'NONE',  ( 93.00000000000000000, 112.2744378736303332, -48.59999999453763309 ) ) ;
#17842=( BOUNDED_CURVE ( )  B_SPLINE_CURVE ( 2, ( #23020, #14302, #18737, #5916, #25017, #14165, #12432, #1779, #25288, #14582, #3634 ),
 .UNSPECIFIED., .F., .F. ) 
 B_SPLINE_CURVE_WITH_KNOTS ( ( 3, 2, 2, 2, 2, 3 ),
 ( 0.000000000000000000, 0.02000000000000000042, 0.04000000000000000083, 0.05999999999999999778, 0.08000000000000000167, 0.1000000000000000194 ),
 .UNSPECIFIED. ) 
 CURVE ( )  GEOMETRIC_REPRESENTATION_ITEM ( )  RATIONAL_B_SPLINE_CURVE ( ( 1.000000000000000000, 0.9510565162951535312, 1.000000000000000000, 0.9510565162951535312, 1.000000000000000000, 0.9510565162951535312, 1.000000000000000000, 0.9510565162951535312, 1.000000000000000000, 0.9510565162951535312, 1.000000000000000000 ) ) 
 REPRESENTATION_ITEM ( '' )  );
#17872=CARTESIAN_POINT ( 'NONE',  ( 108.0825317499999869, 112.6261737610028320, -52.52499999726881441 ) ) ;
#17905=CARTESIAN_POINT ( 'NONE',  ( 104.3262379212492448, 115.9545556584642867, -55.19999999453763451 ) ) ;
#17923=CARTESIAN_POINT ( 'NONE',  ( 94.33688103937535629, 105.8855032339526758, -52.80000000000001137 ) ) ;
#17927=CARTESIAN_POINT ( 'NONE',  ( 92.45873412499997812, 110.0000000000000000, -55.31249999863442213 ) ) ;
#17939=ORIENTED_EDGE ( 'NONE', *, *, #6071, .T. ) ;
#17950=CARTESIAN_POINT ( 'NONE',  ( 97.83688103937537051, 103.3426043859339103, -48.60000000000000853 ) ) ;
#17976=CARTESIAN_POINT ( 'NONE',  ( 93.46109445667489979, 114.7507929638356785, -51.82499999726881867 ) ) ;
#17985=EDGE_LOOP ( 'NONE', ( #8825, #12697, #6833, #25215 ) ) ;
#17989=DIRECTION ( 'NONE',  ( -1.000000000000000000, 0.000000000000000000, 0.000000000000000000 ) ) ;
#17997=VERTEX_POINT ( 'NONE', #13312 ) ;
#18011=CARTESIAN_POINT ( 'NONE',  ( 95.00472066334982912, 116.8754121666685393, -48.17499999726882010 ) ) ;
#18057=CARTESIAN_POINT ( 'NONE',  ( 99.99999999999997158, 118.4984768113314146, -50.37499999726882294 ) ) ;
#18085=CARTESIAN_POINT ( 'NONE',  ( 99.99999999999997158, 117.3602355696678643, -47.50000000000001421 ) ) ;
#18090=CARTESIAN_POINT ( 'NONE',  ( 95.67376207875069838, 104.0454443415356991, -54.70000000000001705 ) ) ;
#18133=CARTESIAN_POINT ( 'NONE',  ( 92.99999999999998579, 112.2744378736303190, -53.10000000000000142 ) ) ;
#18155=CARTESIAN_POINT ( 'NONE',  ( 95.00472066334982912, 103.1245878333314323, -49.57499999726881157 ) ) ;
#18188=CARTESIAN_POINT ( 'NONE',  ( 102.1631189606246153, 116.6573956140660897, -53.09999999453764019 ) ) ;
#18204=CARTESIAN_POINT ( 'NONE',  ( 92.45873412499997812, 110.0000000000000000, -46.18749999590323085 ) ) ;
#18206=CARTESIAN_POINT ( 'NONE',  ( 104.9952793366501567, 103.1245878333314465, -53.17499999726882010 ) ) ;
#18234=AXIS2_PLACEMENT_3D ( 'NONE', #23656, #12927, #23516 ) ;
#18235=CARTESIAN_POINT ( 'NONE',  ( 95.67376207875072680, 115.9545556584642867, -47.30000000000000426 ) ) ;
#18241=CARTESIAN_POINT ( 'NONE',  ( 92.99999999999998579, 110.0000000000000000, -55.00000000000001421 ) ) ;
#18267=CARTESIAN_POINT ( 'NONE',  ( 104.9952793366501567, 103.1245878333314465, -52.92499999726882010 ) ) ;
#18301=CARTESIAN_POINT ( 'NONE',  ( 93.46109445667489979, 114.7507929638356785, -50.07499999726882578 ) ) ;
#18334=CARTESIAN_POINT ( 'NONE',  ( 92.99999999999995737, 112.2744378736303048, -52.59999999453763309 ) ) ;
#18340=CARTESIAN_POINT ( 'NONE',  ( 97.83688103937535629, 116.6573956140660897, -51.40000000000001279 ) ) ;
#18373=CARTESIAN_POINT ( 'NONE',  ( 97.50236033167490746, 117.6869444889999841, -52.27499999726882862 ) ) ;
#18377=CARTESIAN_POINT ( 'NONE',  ( 107.0000000000000000, 110.0000000000000000, -46.00000000000001421 ) ) ;
#18383=CARTESIAN_POINT ( 'NONE',  ( 108.0825317499999869, 112.6261737610028320, -48.52499999726882152 ) ) ;
#18408=CARTESIAN_POINT ( 'NONE',  ( 95.00472066334981491, 103.1245878333314465, -53.32499999726881157 ) ) ;
#18448=CARTESIAN_POINT ( 'NONE',  ( 108.0825317499999869, 107.3738262389971538, -48.97499999726881015 ) ) ;
#18478=CARTESIAN_POINT ( 'NONE',  ( 92.99999999999998579, 110.0000000000000000, -52.49999999453763877 ) ) ;
#18495=CARTESIAN_POINT ( 'NONE',  ( 91.91746824999998466, 110.0000000000000000, -51.87499999726882294 ) ) ;
#18500=CARTESIAN_POINT ( 'NONE',  ( 92.99999999999998579, 107.7255621263696526, -52.90000000000001990 ) ) ;
#18502=CARTESIAN_POINT ( 'NONE',  ( 99.99999999999997158, 117.3602355696678643, -50.99999999453762456 ) ) ;
#18512=CARTESIAN_POINT ( 'NONE',  ( 99.99999999999997158, 102.6397644303321215, -46.50000000000000711 ) ) ;
#18517=CARTESIAN_POINT ( 'NONE',  ( 108.0825317500000011, 110.0000000000000000, -52.87499999726882294 ) ) ;
#18526=CARTESIAN_POINT ( 'NONE',  ( 93.46109445667489979, 114.7507929638356785, -47.82499999726882578 ) ) ;
#18550=CARTESIAN_POINT ( 'NONE',  ( 108.0825317500000011, 110.0000000000000000, -54.62499999726882294 ) ) ;
#18585=CARTESIAN_POINT ( 'NONE',  ( 102.4976396683250783, 102.3130555110000159, -47.27499999726882152 ) ) ;
#18621=CARTESIAN_POINT ( 'NONE',  ( 92.99999999999998579, 110.0000000000000000, -55.00000000000002132 ) ) ;
#18633=CARTESIAN_POINT ( 'NONE',  ( 102.4976396683250783, 102.3130555110000159, -53.27499999726882862 ) ) ;
#18657=CARTESIAN_POINT ( 'NONE',  ( 104.3262379212492448, 115.9545556584642867, -47.19999999453762740 ) ) ;
#18666=CARTESIAN_POINT ( 'NONE',  ( 106.5389055433250860, 114.7507929638356785, -52.42499999726882010 ) ) ;
#18723=CARTESIAN_POINT ( 'NONE',  ( 102.4976396683250783, 102.3130555110000159, -55.27499999726882152 ) ) ;
#18737=CARTESIAN_POINT ( 'NONE',  ( 94.33688103937534208, 114.1144967660473242, -46.69999999453764161 ) ) ;
#18753=CARTESIAN_POINT ( 'NONE',  ( 108.0825317499999869, 107.3738262389971538, -48.72499999726881015 ) ) ;
#18773=CARTESIAN_POINT ( 'NONE',  ( 104.3262379212492448, 115.9545556584642867, -51.19999999453763451 ) ) ;
#18789=CARTESIAN_POINT ( 'NONE',  ( 94.33688103937534208, 114.1144967660473242, -48.69999999453764161 ) ) ;
#18792=CARTESIAN_POINT ( 'NONE',  ( 102.1631189606246295, 103.3426043859339103, -51.89999999453764445 ) ) ;
#18853=CARTESIAN_POINT ( 'NONE',  ( 92.99999999999998579, 110.0000000000000000, -145.0000000000000284 ) ) ;
#18889=VERTEX_POINT ( 'NONE', #11402 ) ;
#18922=CARTESIAN_POINT ( 'NONE',  ( 93.00000000000000000, 107.7255621263696526, -52.39999999453763024 ) ) ;
#18931=CARTESIAN_POINT ( 'NONE',  ( 102.4976396683250783, 117.6869444889999841, -54.22499999726881725 ) ) ;
#18935=ORIENTED_EDGE ( 'NONE', *, *, #14474, .F. ) ;
#18993=CARTESIAN_POINT ( 'NONE',  ( 108.0825317499999869, 107.3738262389971538, -52.97499999726881015 ) ) ;
#18995=ORIENTED_EDGE ( 'NONE', *, *, #22394, .T. ) ;
#19009=( NAMED_UNIT ( * ) SI_UNIT ( $, .STERADIAN. ) SOLID_ANGLE_UNIT ( ) );
#19034=EDGE_LOOP ( 'NONE', ( #7893, #14535, #16229, #5215, #12807, #9011 ) ) ;
#19060=CARTESIAN_POINT ( 'NONE',  ( 104.3262379212492448, 104.0454443415356991, -51.79999999453762882 ) ) ;
#19099=EDGE_CURVE ( 'NONE', #1922, #14596, #24208, .T. ) ;
#19119=VECTOR ( 'NONE', #16464, 1000.000000000000000 ) ;
#19137=CARTESIAN_POINT ( 'NONE',  ( 91.91746824999998466, 110.0000000000000000, -53.87499999726882294 ) ) ;
#19189=LINE ( 'NONE', #23473, #25340 ) ;
#19203=CARTESIAN_POINT ( 'NONE',  ( 99.99999999999997158, 117.3602355696678501, -52.99999999453763166 ) ) ;
#19211=CARTESIAN_POINT ( 'NONE',  ( 108.0825317499999869, 112.6261737610028320, -50.52499999726881441 ) ) ;
#19244=DIRECTION ( 'NONE',  ( 0.000000000000000000, -0.000000000000000000, 1.000000000000000000 ) ) ;
#19275=CARTESIAN_POINT ( 'NONE',  ( 104.9952793366501709, 103.1245878333314323, -49.17499999726881299 ) ) ;
#19280=CARTESIAN_POINT ( 'NONE',  ( 99.99999999999997158, 118.4984768113314004, -54.37499999726880873 ) ) ;
#19283=ORIENTED_EDGE ( 'NONE', *, *, #22394, .F. ) ;
#19332=CARTESIAN_POINT ( 'NONE',  ( 107.0000000000000000, 110.0000000000000000, -45.00000000000000711 ) ) ;
#19337=DIRECTION ( 'NONE',  ( 5.782411586589358625E-17, -0.000000000000000000, 1.000000000000000000 ) ) ;
#19338=CARTESIAN_POINT ( 'NONE',  ( 91.91746824999998466, 110.0000000000000000, -55.87499999726882294 ) ) ;
#19340=CARTESIAN_POINT ( 'NONE',  ( 102.1631189606246153, 116.6573956140660897, -49.09999999453764019 ) ) ;
#19361=CARTESIAN_POINT ( 'NONE',  ( 92.99999999999998579, 110.0000000000000000, -49.00000000000001421 ) ) ;
#19368=CIRCLE ( 'NONE', #5444, 5.000000000000004441 ) ;
#19407=FACE_OUTER_BOUND ( 'NONE', #27619, .T. ) ;
#19408=ORIENTED_EDGE ( 'NONE', *, *, #13516, .F. ) ;
#19431=FACE_OUTER_BOUND ( 'NONE', #3741, .T. ) ;
#19434=ORIENTED_EDGE ( 'NONE', *, *, #13267, .F. ) ;
#19446=CARTESIAN_POINT ( 'NONE',  ( 102.4976396683250783, 117.6869444889999841, -52.22499999726882436 ) ) ;
#19480=DIRECTION ( 'NONE',  ( 5.782411586589358625E-17, -0.000000000000000000, 1.000000000000000000 ) ) ;
#19503=CARTESIAN_POINT ( 'NONE',  ( 99.99999999999997158, 102.6397644303321215, -47.99999999453763877 ) ) ;
#19524=CARTESIAN_POINT ( 'NONE',  ( 93.00000000000000000, 107.7255621263696526, -48.90000000000001279 ) ) ;
#19550=CARTESIAN_POINT ( 'NONE',  ( 97.50236033167490746, 102.3130555110000159, -51.22499999726882436 ) ) ;
#19552=CARTESIAN_POINT ( 'NONE',  ( 99.99999999999997158, 118.4984768113314004, -48.37499999726881583 ) ) ;
#19560=CARTESIAN_POINT ( 'NONE',  ( 102.1631189606246295, 103.3426043859339103, -54.40000000000001279 ) ) ;
#19586=CARTESIAN_POINT ( 'NONE',  ( 95.00472066334982912, 103.1245878333314323, -53.32499999726881157 ) ) ;
#19663=CARTESIAN_POINT ( 'NONE',  ( 104.3262379212492448, 104.0454443415356991, -52.30000000000001847 ) ) ;
#19687=CARTESIAN_POINT ( 'NONE',  ( 108.0825317499999869, 107.3738262389971680, -46.72499999726881015 ) ) ;
#19689=CARTESIAN_POINT ( 'NONE',  ( 99.99999999999997158, 118.4984768113314004, -50.37499999726881583 ) ) ;
#19703=CYLINDRICAL_SURFACE ( 'NONE', #24462, 7.000000000000006217 ) ;
#19713=ORIENTED_EDGE ( 'NONE', *, *, #24515, .F. ) ;
#19723=CARTESIAN_POINT ( 'NONE',  ( 108.0825317500000011, 110.0000000000000000, -50.62499999726882294 ) ) ;
#19774=CARTESIAN_POINT ( 'NONE',  ( 93.46109445667489979, 114.7507929638356785, -48.07499999726882578 ) ) ;
#19780=ORIENTED_EDGE ( 'NONE', *, *, #20172, .F. ) ;
#19785=CARTESIAN_POINT ( 'NONE',  ( 105.6631189606246153, 114.1144967660473242, -45.80000000000001137 ) ) ;
#19805=CARTESIAN_POINT ( 'NONE',  ( 93.00000000000000000, 107.7255621263696526, -52.90000000000001990 ) ) ;
#19809=ADVANCED_FACE ( 'NONE', ( #1964 ), #8926, .F. ) ;
#19830=CARTESIAN_POINT ( 'NONE',  ( 93.46109445667489979, 114.7507929638356785, -47.82499999726882578 ) ) ;
#19832=CARTESIAN_POINT ( 'NONE',  ( 95.00472066334982912, 116.8754121666685393, -52.17499999726881299 ) ) ;
#19848=DIRECTION ( 'NONE',  ( 1.000000000000000000, 0.000000000000000000, 0.000000000000000000 ) ) ;
#19867=CARTESIAN_POINT ( 'NONE',  ( 95.00472066334982912, 116.8754121666685393, -49.92499999726880588 ) ) ;
#19906=CARTESIAN_POINT ( 'NONE',  ( 102.1631189606246153, 116.6573956140660897, -49.60000000000001563 ) ) ;
#19908=VERTEX_POINT ( 'NONE', #19338 ) ;
#19919=CARTESIAN_POINT ( 'NONE',  ( 95.00472066334981491, 116.8754121666685393, -46.17499999726882720 ) ) ;
#19929=CARTESIAN_POINT ( 'NONE',  ( 99.99999999999997158, 117.3602355696678643, -45.50000000000001421 ) ) ;
#19953=CARTESIAN_POINT ( 'NONE',  ( 107.0000000000000000, 107.7255621263696668, -48.10000000000000142 ) ) ;
#19980=CARTESIAN_POINT ( 'NONE',  ( 91.91746824999998466, 110.0000000000000000, -49.62499999726882294 ) ) ;
#19983=CARTESIAN_POINT ( 'NONE',  ( 93.00000000000000000, 107.7255621263696526, -48.39999999453763024 ) ) ;
#19990=CARTESIAN_POINT ( 'NONE',  ( 105.6631189606246153, 114.1144967660473242, -49.29999999453763593 ) ) ;
#20018=CARTESIAN_POINT ( 'NONE',  ( 95.00472066334982912, 103.1245878333314323, -55.32499999726881157 ) ) ;
#20050=CARTESIAN_POINT ( 'NONE',  ( 99.99999999999997158, 117.3602355696678643, -52.99999999453763166 ) ) ;
#20087=EDGE_LOOP ( 'NONE', ( #23853, #22981, #14167, #11897 ) ) ;
#20099=CARTESIAN_POINT ( 'NONE',  ( 102.1631189606246295, 103.3426043859339103, -50.40000000000001279 ) ) ;
#20122=CARTESIAN_POINT ( 'NONE',  ( 102.4976396683250783, 102.3130555110000159, -51.02499999726882152 ) ) ;
#20159=CARTESIAN_POINT ( 'NONE',  ( 97.50236033167490746, 117.6869444889999841, -50.27499999726882152 ) ) ;
#20172=EDGE_CURVE ( 'NONE', #789, #2926, #11617, .T. ) ;
#20179=VERTEX_POINT ( 'NONE', #960 ) ;
#20194=CARTESIAN_POINT ( 'NONE',  ( 102.1631189606246153, 116.6573956140660897, -51.60000000000001563 ) ) ;
#20202=CARTESIAN_POINT ( 'NONE',  ( 102.4976396683250783, 102.3130555110000159, -47.27499999726882152 ) ) ;
#20229=ORIENTED_EDGE ( 'NONE', *, *, #22032, .F. ) ;
#20231=CARTESIAN_POINT ( 'NONE',  ( 94.33688103937534208, 114.1144967660473242, -47.20000000000000995 ) ) ;
#20236=CARTESIAN_POINT ( 'NONE',  ( 91.91746824999998466, 110.0000000000000000, -49.62499999726882294 ) ) ;
#20259=CARTESIAN_POINT ( 'NONE',  ( 97.50236033167490746, 117.6869444889999841, -54.02499999726882862 ) ) ;
#20267=VERTEX_POINT ( 'NONE', #27185 ) ;
#20268=CARTESIAN_POINT ( 'NONE',  ( 107.0000000000000000, 110.0000000000000000, -49.49999999453764588 ) ) ;
#20285=ORIENTED_EDGE ( 'NONE', *, *, #11083, .F. ) ;
#20298=CARTESIAN_POINT ( 'NONE',  ( 102.4976396683250783, 102.3130555110000159, -51.27499999726882152 ) ) ;
#20351=CARTESIAN_POINT ( 'NONE',  ( 104.9952793366501567, 116.8754121666685393, -52.57499999726881867 ) ) ;
#20378=CARTESIAN_POINT ( 'NONE',  ( 93.00000000000000000, 112.2744378736303332, -47.10000000000000853 ) ) ;
#20382=CARTESIAN_POINT ( 'NONE',  ( 95.00472066334982912, 116.8754121666685393, -49.92499999726880588 ) ) ;
#20447=CARTESIAN_POINT ( 'NONE',  ( 91.91746824999998466, 110.0000000000000000, -51.87499999726882294 ) ) ;
#20455=EDGE_LOOP ( 'NONE', ( #17462, #17668, #27534 ) ) ;
#20485=CARTESIAN_POINT ( 'NONE',  ( 107.0000000000000000, 110.0000000000000000, -52.00000000000001421 ) ) ;
#20496=CARTESIAN_POINT ( 'NONE',  ( 108.0825317500000011, 110.0000000000000000, -52.87499999726882294 ) ) ;
#20519=CARTESIAN_POINT ( 'NONE',  ( 99.99999999999997158, 101.5015231886685854, -55.37499999726883004 ) ) ;
#20529=CARTESIAN_POINT ( 'NONE',  ( 104.3262379212492448, 104.0454443415356991, -54.30000000000001137 ) ) ;
#20550=AXIS2_PLACEMENT_3D ( 'NONE', #2197, #28130, #4327 ) ;
#20558=CARTESIAN_POINT ( 'NONE',  ( 99.99999999999998579, 110.0000000000000000, -145.0000000000000284 ) ) ;
#20588=CARTESIAN_POINT ( 'NONE',  ( 106.5389055433250860, 114.7507929638356785, -52.67499999726882010 ) ) ;
#20592=CARTESIAN_POINT ( 'NONE',  ( 99.99999999999997158, 117.3602355696678501, -45.50000000000001421 ) ) ;
#20635=CARTESIAN_POINT ( 'NONE',  ( 97.50236033167490746, 102.3130555110000159, -51.47499999726882436 ) ) ;
#20639=CARTESIAN_POINT ( 'NONE',  ( 102.1631189606246295, 103.3426043859339103, -52.40000000000001279 ) ) ;
#20659=CARTESIAN_POINT ( 'NONE',  ( 97.50236033167490746, 117.6869444889999841, -54.27499999726882862 ) ) ;
#20670=CARTESIAN_POINT ( 'NONE',  ( 95.67376207875069838, 115.9545556584642867, -53.30000000000000426 ) ) ;
#20695=CARTESIAN_POINT ( 'NONE',  ( 97.50236033167490746, 102.3130555110000159, -55.22499999726881725 ) ) ;
#20723=CARTESIAN_POINT ( 'NONE',  ( 99.99999999999998579, 110.0000000000000000, -45.00000000000000711 ) ) ;
#20729=CARTESIAN_POINT ( 'NONE',  ( 104.9952793366501709, 103.1245878333314323, -49.17499999726881299 ) ) ;
#20771=CARTESIAN_POINT ( 'NONE',  ( 102.4976396683250783, 117.6869444889999841, -52.47499999726882436 ) ) ;
#20793=CARTESIAN_POINT ( 'NONE',  ( 102.1631189606246295, 103.3426043859339103, -46.40000000000001279 ) ) ;
#20797=CARTESIAN_POINT ( 'NONE',  ( 104.9952793366501709, 116.8754121666685393, -52.57499999726881867 ) ) ;
#20805=CARTESIAN_POINT ( 'NONE',  ( 95.00472066334982912, 116.8754121666685393, -45.92499999726882720 ) ) ;
#20848=CARTESIAN_POINT ( 'NONE',  ( 107.0000000000000000, 110.0000000000000000, -54.00000000000001421 ) ) ;
#20866=CARTESIAN_POINT ( 'NONE',  ( 91.91746824999997045, 107.3738262389971538, -53.77499999726881441 ) ) ;
#20868=EDGE_LOOP ( 'NONE', ( #20229, #27817 ) ) ;
#20872=AXIS2_PLACEMENT_3D ( 'NONE', #9934, #12475, #25334 ) ;
#20880=( BOUNDED_CURVE ( )  B_SPLINE_CURVE ( 2, ( #12552, #12418, #14978, #16719, #21003, #14697, #10139, #23697, #21278, #27976, #10426 ),
 .UNSPECIFIED., .F., .T. ) 
 B_SPLINE_CURVE_WITH_KNOTS ( ( 3, 2, 2, 2, 2, 3 ),
 ( 0.6999999999999998446, 0.7199999999999998623, 0.7399999999999998801, 0.7600000000000000089, 0.7800000000000000266, 0.8000000000000000444 ),
 .UNSPECIFIED. ) 
 CURVE ( )  GEOMETRIC_REPRESENTATION_ITEM ( )  RATIONAL_B_SPLINE_CURVE ( ( 1.000000000000000222, 0.9510565162951533091, 1.000000000000000000, 0.9510565162951535312, 1.000000000000000000, 0.9510565162951535312, 1.000000000000000000, 0.9510565162951535312, 1.000000000000000000, 0.9510565162951535312, 1.000000000000000000 ) ) 
 REPRESENTATION_ITEM ( '' )  );
#20910=DIRECTION ( 'NONE',  ( 0.8660254037844392627, 0.000000000000000000, -0.4999999999999987788 ) ) ;
#20934=CARTESIAN_POINT ( 'NONE',  ( 104.3262379212492448, 104.0454443415356991, -49.79999999453762882 ) ) ;
#20944=CARTESIAN_POINT ( 'NONE',  ( 108.0825317499999869, 112.6261737610028320, -52.52499999726881441 ) ) ;
#20992=CARTESIAN_POINT ( 'NONE',  ( 107.0000000000000000, 110.0000000000000000, -50.00000000000000711 ) ) ;
#21003=CARTESIAN_POINT ( 'NONE',  ( 102.1631189606246295, 103.3426043859339103, -53.89999999453763735 ) ) ;
#21009=VERTEX_POINT ( 'NONE', #18377 ) ;
#21015=VERTEX_POINT ( 'NONE', #863 ) ;
#21034=CARTESIAN_POINT ( 'NONE',  ( 97.50236033167490746, 117.6869444889999841, -48.02499999726882152 ) ) ;
#21035=ORIENTED_EDGE ( 'NONE', *, *, #25847, .F. ) ;
#21070=CARTESIAN_POINT ( 'NONE',  ( 99.99999999999998579, 110.0000000000000000, -145.0000000000000284 ) ) ;
#21071=CARTESIAN_POINT ( 'NONE',  ( 104.3262379212492448, 115.9545556584642867, -49.19999999453763451 ) ) ;
#21079=CARTESIAN_POINT ( 'NONE',  ( 91.91746824999998466, 110.0000000000000000, -55.62499999726882294 ) ) ;
#21111=ORIENTED_EDGE ( 'NONE', *, *, #21157, .T. ) ;
#21139=CARTESIAN_POINT ( 'NONE',  ( 104.9952793366501709, 103.1245878333314323, -55.17499999726882720 ) ) ;
#21157=EDGE_CURVE ( 'NONE', #2581, #16704, #12524, .T. ) ;
#21169=DIRECTION ( 'NONE',  ( -5.782411586589357392E-17, 0.000000000000000000, -1.000000000000000000 ) ) ;
#21209=CARTESIAN_POINT ( 'NONE',  ( 92.99999999999998579, 110.0000000000000000, -50.49999999453763877 ) ) ;
#21218=CARTESIAN_POINT ( 'NONE',  ( 95.00472066334982912, 103.1245878333314323, -55.32499999726881157 ) ) ;
#21240=CYLINDRICAL_SURFACE ( 'NONE', #18234, 7.000000000000006217 ) ;
#21250=CARTESIAN_POINT ( 'NONE',  ( 102.1631189606246153, 116.6573956140660897, -45.60000000000001563 ) ) ;
#21278=CARTESIAN_POINT ( 'NONE',  ( 94.33688103937535629, 105.8855032339526758, -54.29999999453764303 ) ) ;
#21281=CARTESIAN_POINT ( 'NONE',  ( 97.50236033167490746, 102.3130555110000159, -53.47499999726882436 ) ) ;
#21293=VECTOR ( 'NONE', #4007, 1000.000000000000000 ) ;
#21309=CARTESIAN_POINT ( 'NONE',  ( 102.4976396683250783, 102.3130555110000159, -47.02499999726882152 ) ) ;
#21352=CARTESIAN_POINT ( 'NONE',  ( 92.99999999999998579, 110.0000000000000000, -54.49999999453763877 ) ) ;
#21355=CARTESIAN_POINT ( 'NONE',  ( 99.99999999999997158, 102.6397644303321215, -51.99999999453763877 ) ) ;
#21361=CARTESIAN_POINT ( 'NONE',  ( 108.0825317500000011, 110.0000000000000000, -54.62499999726882294 ) ) ;
#21369=CARTESIAN_POINT ( 'NONE',  ( 99.99999999999998579, 110.0000000000000000, -145.0000000000000284 ) ) ;
#21372=LINE ( 'NONE', #12914, #14505 ) ;
#21390=ORIENTED_EDGE ( 'NONE', *, *, #2971, .T. ) ;
#21395=CARTESIAN_POINT ( 'NONE',  ( 99.99999999999997158, 102.6397644303321215, -46.50000000000001421 ) ) ;
#21421=CARTESIAN_POINT ( 'NONE',  ( 108.0825317500000011, 110.0000000000000000, -46.87499999726882294 ) ) ;
#21427=VECTOR ( 'NONE', #1749, 1000.000000000000000 ) ;
#21431=DIRECTION ( 'NONE',  ( 0.000000000000000000, -1.000000000000000000, 0.000000000000000000 ) ) ;
#21454=CARTESIAN_POINT ( 'NONE',  ( 91.91746824999998466, 110.0000000000000000, -45.62499999726882294 ) ) ;
#21485=CARTESIAN_POINT ( 'NONE',  ( 107.0000000000000000, 107.7255621263696668, -53.59999999453763309 ) ) ;
#21488=CARTESIAN_POINT ( 'NONE',  ( 94.33688103937535629, 105.8855032339526758, -56.29999999453763593 ) ) ;
#21493=CARTESIAN_POINT ( 'NONE',  ( 93.46109445667489979, 105.2492070361643215, -51.42499999726882010 ) ) ;
#21496=EDGE_LOOP ( 'NONE', ( #19283, #13077, #3377, #18935 ) ) ;
#21499=CYLINDRICAL_SURFACE ( 'NONE', #3307, 7.000000000000006217 ) ;
#21506=CARTESIAN_POINT ( 'NONE',  ( 97.83688103937537051, 103.3426043859339103, -48.60000000000000853 ) ) ;
#21529=APPLICATION_CONTEXT ( 'automotive_design' ) ;
#21559=CARTESIAN_POINT ( 'NONE',  ( 108.0825317499999869, 112.6261737610028320, -46.77499999726882152 ) ) ;
#21560=ORIENTED_EDGE ( 'NONE', *, *, #6927, .T. ) ;
#21577=CYLINDRICAL_SURFACE ( 'NONE', #20550, 7.000000000000006217 ) ;
#21591=CARTESIAN_POINT ( 'NONE',  ( 93.46109445667489979, 114.7507929638356785, -51.82499999726881867 ) ) ;
#21627=LINE ( 'NONE', #24319, #14940 ) ;
#21628=CARTESIAN_POINT ( 'NONE',  ( 95.67376207875072680, 115.9545556584642867, -49.30000000000000426 ) ) ;
#21670=CARTESIAN_POINT ( 'NONE',  ( 92.99999999999998579, 110.0000000000000000, -49.00000000000001421 ) ) ;
#21698=CARTESIAN_POINT ( 'NONE',  ( 95.00472066334981491, 103.1245878333314465, -47.32499999726881867 ) ) ;
#21700=CARTESIAN_POINT ( 'NONE',  ( 91.91746824999997045, 112.6261737610028320, -45.97499999726882436 ) ) ;
#21728=ORIENTED_EDGE ( 'NONE', *, *, #24502, .F. ) ;
#21738=CARTESIAN_POINT ( 'NONE',  ( 93.46109445667489979, 105.2492070361643215, -53.42499999726882720 ) ) ;
#21772=CARTESIAN_POINT ( 'NONE',  ( 99.99999999999997158, 117.3602355696678643, -54.99999999453763166 ) ) ;
#21785=CARTESIAN_POINT ( 'NONE',  ( 97.50236033167490746, 102.3130555110000159, -49.47499999726882436 ) ) ;
#21791=CARTESIAN_POINT ( 'NONE',  ( 104.3262379212492448, 104.0454443415356991, -47.79999999453763593 ) ) ;
#21817=CARTESIAN_POINT ( 'NONE',  ( 107.0000000000000000, 112.2744378736303332, -51.90000000000000568 ) ) ;
#21825=UNCERTAINTY_MEASURE_WITH_UNIT (LENGTH_MEASURE( 1.000000000000000082E-05 ), #8294, 'distance_accuracy_value', 'NONE');
#21840=DIRECTION ( 'NONE',  ( -5.782411586589357392E-17, 0.000000000000000000, -1.000000000000000000 ) ) ;
#21842=CARTESIAN_POINT ( 'NONE',  ( 99.99999999999997158, 101.5015231886685712, -49.12499999726882294 ) ) ;
#21844=CARTESIAN_POINT ( 'NONE',  ( 97.50236033167490746, 117.6869444889999841, -50.27499999726882152 ) ) ;
#21879=CARTESIAN_POINT ( 'NONE',  ( 93.46109445667489979, 105.2492070361643215, -51.42499999726882010 ) ) ;
#21916=CARTESIAN_POINT ( 'NONE',  ( 94.33688103937534208, 114.1144967660473242, -54.69999999453764161 ) ) ;
#21919=ORIENTED_EDGE ( 'NONE', *, *, #11787, .T. ) ;
#21920=CARTESIAN_POINT ( 'NONE',  ( 104.3262379212492448, 104.0454443415356991, -55.79999999453763593 ) ) ;
#21928=CARTESIAN_POINT ( 'NONE',  ( 93.46109445667489979, 114.7507929638356785, -46.07499999726881867 ) ) ;
#21954=CARTESIAN_POINT ( 'NONE',  ( 92.99999999999998579, 110.0000000000000000, -51.00000000000000711 ) ) ;
#21976=DIRECTION ( 'NONE',  ( -1.000000000000000000, 0.000000000000000000, 0.000000000000000000 ) ) ;
#21978=CARTESIAN_POINT ( 'NONE',  ( 93.46109445667489979, 105.2492070361643215, -49.42499999726882010 ) ) ;
#21980=CARTESIAN_POINT ( 'NONE',  ( 93.46109445667489979, 105.2492070361643215, -51.67499999726882010 ) ) ;
#22013=CARTESIAN_POINT ( 'NONE',  ( 97.50236033167490746, 117.6869444889999841, -54.02499999726882862 ) ) ;
#22032=EDGE_CURVE ( 'NONE', #11248, #3337, #24424, .T. ) ;
#22054=ORIENTED_EDGE ( 'NONE', *, *, #15930, .F. ) ;
#22055=CARTESIAN_POINT ( 'NONE',  ( 95.67376207875072680, 104.0454443415356991, -56.19999999453762740 ) ) ;
#22066=CARTESIAN_POINT ( 'NONE',  ( 102.4976396683250783, 117.6869444889999841, -48.47499999726882436 ) ) ;
#22074=CARTESIAN_POINT ( 'NONE',  ( 97.83688103937537051, 103.3426043859339103, -48.09999999453764019 ) ) ;
#22076=CARTESIAN_POINT ( 'NONE',  ( 95.67376207875072680, 115.9545556584642867, -45.30000000000000426 ) ) ;
#22096=CARTESIAN_POINT ( 'NONE',  ( 102.1631189606246153, 116.6573956140660897, -49.60000000000001563 ) ) ;
#22120=CARTESIAN_POINT ( 'NONE',  ( 108.0825317500000011, 110.0000000000000000, -46.62499999726882294 ) ) ;
#22122=CARTESIAN_POINT ( 'NONE',  ( 102.1631189606246153, 116.6573956140660897, -47.09999999453764019 ) ) ;
#22157=CARTESIAN_POINT ( 'NONE',  ( 91.91746824999997045, 107.3738262389971538, -53.52499999726882862 ) ) ;
#22189=CARTESIAN_POINT ( 'NONE',  ( 92.99999999999998579, 112.2744378736303190, -54.59999999453764019 ) ) ;
#22200=ORIENTED_EDGE ( 'NONE', *, *, #4590, .F. ) ;
#22238=CARTESIAN_POINT ( 'NONE',  ( 105.6631189606246153, 114.1144967660473242, -49.80000000000001137 ) ) ;
#22264=CARTESIAN_POINT ( 'NONE',  ( 108.0825317499999869, 112.6261737610028320, -50.52499999726881441 ) ) ;
#22266=CARTESIAN_POINT ( 'NONE',  ( 92.99999999999998579, 110.0000000000000000, -46.49999999453763877 ) ) ;
#22267=ORIENTED_EDGE ( 'NONE', *, *, #1710, .F. ) ;
#22300=CARTESIAN_POINT ( 'NONE',  ( 91.91746824999997045, 112.6261737610028320, -49.97499999726881725 ) ) ;
#22347=CARTESIAN_POINT ( 'NONE',  ( 91.91746824999997045, 112.6261737610028320, -45.97499999726882436 ) ) ;
#22376=CARTESIAN_POINT ( 'NONE',  ( 106.5389055433250860, 105.2492070361643215, -46.82499999726881867 ) ) ;
#22394=EDGE_CURVE ( 'NONE', #20179, #18889, #5071, .T. ) ;
#22402=CARTESIAN_POINT ( 'NONE',  ( 91.91746824999997045, 112.6261737610028320, -53.72499999726881725 ) ) ;
#22414=ORIENTED_EDGE ( 'NONE', *, *, #8600, .T. ) ;
#22442=CARTESIAN_POINT ( 'NONE',  ( 108.0825317499999869, 112.6261737610028320, -46.77499999726882152 ) ) ;
#22446=ORIENTED_EDGE ( 'NONE', *, *, #15415, .T. ) ;
#22488=CARTESIAN_POINT ( 'NONE',  ( 95.00472066334981491, 103.1245878333314465, -55.57499999726882578 ) ) ;
#22512=PRODUCT_DEFINITION ( 'UNKNOWN', '', #10832, #10044 ) ;
#22521=CARTESIAN_POINT ( 'NONE',  ( 104.9952793366501709, 116.8754121666685393, -46.32499999726881867 ) ) ;
#22546=CARTESIAN_POINT ( 'NONE',  ( 99.99999999999997158, 101.5015231886685712, -55.12499999726881583 ) ) ;
#22551=EDGE_CURVE ( 'NONE', #20179, #789, #27511, .T. ) ;
#22584=EDGE_CURVE ( 'NONE', #17997, #9015, #23092, .T. ) ;
#22586=CARTESIAN_POINT ( 'NONE',  ( 93.46109445667489979, 105.2492070361643215, -47.67499999726882720 ) ) ;
#22587=ORIENTED_EDGE ( 'NONE', *, *, #8245, .F. ) ;
#22610=LINE ( 'NONE', #11884, #12953 ) ;
#22622=ORIENTED_EDGE ( 'NONE', *, *, #25863, .F. ) ;
#22636=CARTESIAN_POINT ( 'NONE',  ( 99.99999999999997158, 101.5015231886685712, -55.37499999726881583 ) ) ;
#22661=DIRECTION ( 'NONE',  ( 1.000000000000000000, 0.000000000000000000, 0.000000000000000000 ) ) ;
#22666=CARTESIAN_POINT ( 'NONE',  ( 99.99999999999997158, 101.5015231886685854, -47.12499999726882294 ) ) ;
#22691=CARTESIAN_POINT ( 'NONE',  ( 95.00472066334981491, 116.8754121666685393, -53.92499999726882720 ) ) ;
#22728=CARTESIAN_POINT ( 'NONE',  ( 102.4976396683250783, 117.6869444889999841, -52.47499999726882436 ) ) ;
#22755=ADVANCED_FACE ( 'NONE', ( #15059 ), #21499, .T. ) ;
#22781=CARTESIAN_POINT ( 'NONE',  ( 106.9999999999999858, 107.7255621263696810, -52.10000000000000142 ) ) ;
#22783=CARTESIAN_POINT ( 'NONE',  ( 97.83688103937535629, 116.6573956140660897, -50.89999999453764445 ) ) ;
#22785=LINE ( 'NONE', #11352, #26052 ) ;
#22800=CARTESIAN_POINT ( 'NONE',  ( 105.6631189606246295, 105.8855032339526758, -47.69999999453764161 ) ) ;
#22809=CARTESIAN_POINT ( 'NONE',  ( 97.50236033167490746, 102.3130555110000159, -49.22499999726882436 ) ) ;
#22828=CYLINDRICAL_SURFACE ( 'NONE', #5022, 7.000000000000006217 ) ;
#22867=CARTESIAN_POINT ( 'NONE',  ( 99.99999999999997158, 118.4984768113314004, -48.37499999726881583 ) ) ;
#22871=VERTEX_POINT ( 'NONE', #1849 ) ;
#22901=ORIENTED_EDGE ( 'NONE', *, *, #10885, .F. ) ;
#22914=CARTESIAN_POINT ( 'NONE',  ( 95.00472066334981491, 103.1245878333314465, -51.57499999726881157 ) ) ;
#22927=CARTESIAN_POINT ( 'NONE',  ( 105.6631189606246295, 105.8855032339526758, -49.69999999453764161 ) ) ;
#22939=CARTESIAN_POINT ( 'NONE',  ( 91.91746824999997045, 107.3738262389971538, -51.77499999726881441 ) ) ;
#22950=CARTESIAN_POINT ( 'NONE',  ( 102.4976396683250783, 117.6869444889999841, -48.22499999726881725 ) ) ;
#22974=CARTESIAN_POINT ( 'NONE',  ( 106.5389055433250860, 114.7507929638356785, -54.42499999726882720 ) ) ;
#22981=ORIENTED_EDGE ( 'NONE', *, *, #11405, .F. ) ;
#23020=CARTESIAN_POINT ( 'NONE',  ( 92.99999999999998579, 110.0000000000000000, -46.49999999453763877 ) ) ;
#23051=CARTESIAN_POINT ( 'NONE',  ( 93.46109445667489979, 105.2492070361643215, -53.67499999726882720 ) ) ;
#23074=CARTESIAN_POINT ( 'NONE',  ( 108.0825317499999869, 112.6261737610028320, -54.77499999726881441 ) ) ;
#23084=CARTESIAN_POINT ( 'NONE',  ( 91.91746824999997045, 107.3738262389971538, -53.52499999726882862 ) ) ;
#23086=ORIENTED_EDGE ( 'NONE', *, *, #24515, .T. ) ;
#23092=LINE ( 'NONE', #1575, #642 ) ;
#23175=FACE_OUTER_BOUND ( 'NONE', #26663, .T. ) ;
#23203=CARTESIAN_POINT ( 'NONE',  ( 102.1631189606246295, 103.3426043859339103, -49.89999999453763735 ) ) ;
#23214=CARTESIAN_POINT ( 'NONE',  ( 105.6631189606246295, 105.8855032339526758, -51.69999999453764161 ) ) ;
#23217=CARTESIAN_POINT ( 'NONE',  ( 105.6631189606246295, 105.8855032339526758, -51.69999999453764161 ) ) ;
#23223=CARTESIAN_POINT ( 'NONE',  ( 104.9952793366501709, 116.8754121666685393, -54.32499999726881867 ) ) ;
#23272=CARTESIAN_POINT ( 'NONE',  ( 94.33688103937535629, 105.8855032339526758, -50.80000000000001137 ) ) ;
#23285=CARTESIAN_POINT ( 'NONE',  ( 106.5389055433250860, 105.2492070361643215, -55.07499999726882578 ) ) ;
#23314=CARTESIAN_POINT ( 'NONE',  ( 99.99999999999997158, 118.4984768113314004, -46.12499999726880873 ) ) ;
#23349=CARTESIAN_POINT ( 'NONE',  ( 107.0000000000000000, 112.2744378736303332, -53.39999999453764445 ) ) ;
#23351=ORIENTED_EDGE ( 'NONE', *, *, #6697, .T. ) ;
#23357=CARTESIAN_POINT ( 'NONE',  ( 99.99999999999997158, 118.4984768113314004, -54.12499999726881583 ) ) ;
#23365=DIRECTION ( 'NONE',  ( 5.782411586589358625E-17, -0.000000000000000000, 1.000000000000000000 ) ) ;
#23383=DIRECTION ( 'NONE',  ( -5.782411586589357392E-17, 0.000000000000000000, -1.000000000000000000 ) ) ;
#23429=AXIS2_PLACEMENT_3D ( 'NONE', #9744, #12805, #19244 ) ;
#23449=CARTESIAN_POINT ( 'NONE',  ( 104.9952793366501709, 103.1245878333314323, -46.92499999726882010 ) ) ;
#23450=ADVANCED_FACE ( 'NONE', ( #26157, #6625 ), #25881, .F. ) ;
#23473=CARTESIAN_POINT ( 'NONE',  ( 92.99999999999998579, 110.0000000000000000, -145.0000000000000284 ) ) ;
#23485=CARTESIAN_POINT ( 'NONE',  ( 102.1631189606246295, 103.3426043859339103, -49.89999999453763735 ) ) ;
#23494=CARTESIAN_POINT ( 'NONE',  ( 108.0825317499999869, 107.3738262389971538, -50.72499999726881015 ) ) ;
#23516=DIRECTION ( 'NONE',  ( 1.000000000000000000, 0.000000000000000000, 0.000000000000000000 ) ) ;
#23526=CARTESIAN_POINT ( 'NONE',  ( 107.0000000000000000, 110.0000000000000000, -46.00000000000001421 ) ) ;
#23546=CYLINDRICAL_SURFACE ( 'NONE', #16711, 7.000000000000006217 ) ;
#23554=CARTESIAN_POINT ( 'NONE',  ( 95.00472066334982912, 103.1245878333314323, -49.57499999726881157 ) ) ;
#23584=CARTESIAN_POINT ( 'NONE',  ( 97.50236033167490746, 102.3130555110000159, -47.22499999726881725 ) ) ;
#23598=DIRECTION ( 'NONE',  ( -5.782411586589357392E-17, 0.000000000000000000, -1.000000000000000000 ) ) ;
#23608=DIRECTION ( 'NONE',  ( 1.000000000000000000, 0.000000000000000000, 0.000000000000000000 ) ) ;
#23626=CARTESIAN_POINT ( 'NONE',  ( 99.99999999999997158, 102.6397644303321215, -49.99999999453764588 ) ) ;
#23635=CARTESIAN_POINT ( 'NONE',  ( 91.91746824999998466, 110.0000000000000000, -51.62499999726882294 ) ) ;
#23648=CARTESIAN_POINT ( 'NONE',  ( 107.0000000000000142, 107.7255621263696668, -48.10000000000001563 ) ) ;
#23656=CARTESIAN_POINT ( 'NONE',  ( 99.99999999999998579, 110.0000000000000000, -145.0000000000000284 ) ) ;
#23665=VERTEX_POINT ( 'NONE', #13593 ) ;
#23666=VECTOR ( 'NONE', #7125, 1000.000000000000114 ) ;
#23667=FACE_OUTER_BOUND ( 'NONE', #25279, .T. ) ;
#23672=ORIENTED_EDGE ( 'NONE', *, *, #4590, .T. ) ;
#23694=CARTESIAN_POINT ( 'NONE',  ( 108.0825317499999869, 112.6261737610028320, -50.77499999726882152 ) ) ;
#23697=CARTESIAN_POINT ( 'NONE',  ( 95.67376207875072680, 104.0454443415356991, -54.19999999453764872 ) ) ;
#23708=FACE_OUTER_BOUND ( 'NONE', #27224, .T. ) ;
#23715=ORIENTED_EDGE ( 'NONE', *, *, #8047, .T. ) ;
#23719=SURFACE_STYLE_FILL_AREA ( #8320 ) ;
#23729=CARTESIAN_POINT ( 'NONE',  ( 108.0825317499999869, 112.6261737610028320, -48.52499999726882152 ) ) ;
#23753=LINE ( 'NONE', #6636, #12637 ) ;
#23759=DIRECTION ( 'NONE',  ( 1.000000000000000000, 0.000000000000000000, 0.000000000000000000 ) ) ;
#23761=CARTESIAN_POINT ( 'NONE',  ( 95.67376207875069838, 115.9545556584642867, -48.79999999453764303 ) ) ;
#23802=CARTESIAN_POINT ( 'NONE',  ( 102.1631189606246153, 116.6573956140660897, -51.60000000000001563 ) ) ;
#23830=CARTESIAN_POINT ( 'NONE',  ( 97.50236033167490746, 102.3130555110000159, -47.47499999726881725 ) ) ;
#23849=CARTESIAN_POINT ( 'NONE',  ( 94.99999999999998579, 110.0000000000000000, -45.00000000000000711 ) ) ;
#23853=ORIENTED_EDGE ( 'NONE', *, *, #22551, .F. ) ;
#23855=( NAMED_UNIT ( * ) SI_UNIT ( $, .STERADIAN. ) SOLID_ANGLE_UNIT ( ) );
#23864=CARTESIAN_POINT ( 'NONE',  ( 104.9952793366501709, 103.1245878333314323, -54.92499999726882720 ) ) ;
#23912=CARTESIAN_POINT ( 'NONE',  ( 104.9952793366501567, 103.1245878333314465, -49.17499999726881299 ) ) ;
#23944=CARTESIAN_POINT ( 'NONE',  ( 97.83688103937535629, 116.6573956140660897, -51.40000000000001279 ) ) ;
#23970=CARTESIAN_POINT ( 'NONE',  ( 104.9952793366501567, 116.8754121666685393, -46.32499999726881867 ) ) ;
#23973=CARTESIAN_POINT ( 'NONE',  ( 91.91746824999997045, 112.6261737610028320, -49.97499999726881725 ) ) ;
#24009=CARTESIAN_POINT ( 'NONE',  ( 99.99999999999997158, 101.5015231886685854, -51.12499999726882294 ) ) ;
#24028=DIRECTION ( 'NONE',  ( 0.000000000000000000, 0.000000000000000000, 1.000000000000000000 ) ) ;
#24055=CARTESIAN_POINT ( 'NONE',  ( 91.91746824999997045, 107.3738262389971680, -47.77499999726881441 ) ) ;
#24064=APPLICATION_CONTEXT ( 'automotive_design' ) ;
#24086=CARTESIAN_POINT ( 'NONE',  ( 93.00000000000000000, 107.7255621263696526, -50.90000000000001990 ) ) ;
#24109=CARTESIAN_POINT ( 'NONE',  ( 93.46109445667489979, 105.2492070361643215, -51.42499999726882010 ) ) ;
#24112=CARTESIAN_POINT ( 'NONE',  ( 95.00472066334982912, 103.1245878333314323, -51.57499999726880446 ) ) ;
#24121=VERTEX_POINT ( 'NONE', #23849 ) ;
#24149=CARTESIAN_POINT ( 'NONE',  ( 104.9952793366501709, 116.8754121666685393, -54.32499999726881867 ) ) ;
#24184=CARTESIAN_POINT ( 'NONE',  ( 95.67376207875069838, 104.0454443415356991, -56.19999999453762740 ) ) ;
#24208=( BOUNDED_CURVE ( )  B_SPLINE_CURVE ( 2, ( #25679, #12694, #10563, #8429, #17118, #8574, #26250, #23970, #24390, #6994, #22120, #19687, #24535, #13392, #5020, #26537, #2738, #21698, #31, #6710, #6852, #24249, #19830, #13246, #15252, #15541, #9140, #2599, #4449, #11260, #13103, #17405, #15397, #2173, #10835, #21842, #2454, #8713, #21978, #26397, #19980, #26105, #4732, #15688, #458, #11116, #13542, #17833, #4878, #22264, #11403, #6570, #315, #9002, #20122, #17694, #19550, #600, #24109, #9279, #17547, #2318, #17976, #26685, #10975, #174, #4586, #7132, #15829, #8856, #3015, #16405, #7713, #18267, #5302, #13685, #11831, #18408, #26832, #14253, #3302, #22402, #5159, #22691, #20259, #13966, #27115, #11972, #22974, #1036, #18550, #27254, #3161, #5588, #25102, #22546, #20695, #9418, #14112, #25236, #11684 ),
 .UNSPECIFIED., .F., .F. ) 
 B_SPLINE_CURVE_WITH_KNOTS ( ( 3, 2, 2, 2, 2, 2, 2, 2, 2, 2, 2, 2, 2, 2, 2, 2, 2, 2, 2, 2, 2, 2, 2, 2, 2, 2, 2, 2, 2, 2, 2, 2, 2, 2, 2, 2, 2, 2, 2, 2, 2, 2, 2, 2, 2, 2, 2, 2, 2, 2, 3 ),
 ( 0.000000000000000000, 0.02000000000000000042, 0.04000000000000000083, 0.05999999999999999778, 0.08000000000000000167, 0.1000000000000000056, 0.1199999999999999956, 0.1400000000000000133, 0.1600000000000000033, 0.1799999999999999933, 0.2000000000000000111, 0.2200000000000000011, 0.2399999999999999911, 0.2600000000000000089, 0.2800000000000000266, 0.2999999999999999889, 0.3200000000000000067, 0.3400000000000000244, 0.3599999999999999867, 0.3800000000000000044, 0.4000000000000000222, 0.4199999999999999845, 0.4400000000000000022, 0.4600000000000000200, 0.4799999999999999822, 0.5000000000000000000, 0.5200000000000000178, 0.5400000000000000355, 0.5600000000000000533, 0.5799999999999999600, 0.5999999999999999778, 0.6199999999999999956, 0.6400000000000000133, 0.6600000000000000311, 0.6800000000000000488, 0.6999999999999999556, 0.7199999999999999734, 0.7399999999999999911, 0.7600000000000000089, 0.7800000000000000266, 0.8000000000000000444, 0.8199999999999999512, 0.8399999999999999689, 0.8599999999999999867, 0.8800000000000000044, 0.9000000000000000222, 0.9200000000000000400, 0.9399999999999999467, 0.9599999999999999645, 0.9799999999999999822, 1.000000000000000000 ),
 .UNSPECIFIED. ) 
 CURVE ( )  GEOMETRIC_REPRESENTATION_ITEM ( )  RATIONAL_B_SPLINE_CURVE ( ( 1.000000000000000000, 0.9510565162951535312, 1.000000000000000000, 0.9510565162951535312, 1.000000000000000000, 0.9510565162951535312, 1.000000000000000000, 0.9510565162951535312, 1.000000000000000000, 0.9510565162951535312, 1.000000000000000000, 0.9510565162951535312, 1.000000000000000000, 0.9510565162951535312, 1.000000000000000000, 0.9510565162951535312, 1.000000000000000000, 0.9510565162951535312, 1.000000000000000000, 0.9510565162951535312, 1.000000000000000000, 0.9510565162951535312, 1.000000000000000000, 0.9510565162951535312, 1.000000000000000000, 0.9510565162951535312, 1.000000000000000000, 0.9510565162951535312, 1.000000000000000000, 0.9510565162951535312, 1.000000000000000000, 0.9510565162951535312, 1.000000000000000000, 0.9510565162951535312, 1.000000000000000000, 0.9510565162951535312, 1.000000000000000000, 0.9510565162951535312, 1.000000000000000000, 0.9510565162951535312, 1.000000000000000000, 0.9510565162951535312, 1.000000000000000000, 0.9510565162951535312, 1.000000000000000000, 0.9510565162951535312, 1.000000000000000000, 0.9510565162951535312, 1.000000000000000000, 0.9510565162951535312, 1.000000000000000000, 0.9510565162951535312, 1.000000000000000000, 0.9510565162951535312, 1.000000000000000000, 0.9510565162951535312, 1.000000000000000000, 0.9510565162951535312, 1.000000000000000000, 0.9510565162951535312, 1.000000000000000000, 0.9510565162951535312, 1.000000000000000000, 0.9510565162951535312, 1.000000000000000000, 0.9510565162951535312, 1.000000000000000000, 0.9510565162951535312, 1.000000000000000000, 0.9510565162951535312, 1.000000000000000000, 0.9510565162951535312, 1.000000000000000000, 0.9510565162951535312, 1.000000000000000000, 0.9510565162951535312, 1.000000000000000000, 0.9510565162951535312, 1.000000000000000000, 0.9510565162951535312, 1.000000000000000000, 0.9510565162951535312, 1.000000000000000000, 0.9510565162951535312, 1.000000000000000000, 0.9510565162951535312, 1.000000000000000000, 0.9510565162951535312, 1.000000000000000000, 0.9510565162951535312, 1.000000000000000000, 0.9510565162951535312, 1.000000000000000000, 0.9510565162951535312, 1.000000000000000000, 0.9510565162951535312, 1.000000000000000000, 0.9510565162951535312, 1.000000000000000000, 0.9510565162951535312, 1.000000000000000000 ) ) 
 REPRESENTATION_ITEM ( '' )  );
#24226=CARTESIAN_POINT ( 'NONE',  ( 95.67376207875069838, 104.0454443415356991, -48.70000000000000995 ) ) ;
#24249=CARTESIAN_POINT ( 'NONE',  ( 91.91746824999997045, 112.6261737610028320, -47.72499999726881725 ) ) ;
#24252=CARTESIAN_POINT ( 'NONE',  ( 104.9952793366501709, 116.8754121666685393, -54.57499999726882578 ) ) ;
#24253=EDGE_LOOP ( 'NONE', ( #15620, #23715 ) ) ;
#24261=CARTESIAN_POINT ( 'NONE',  ( 104.3262379212492448, 115.9545556584642867, -49.19999999453763451 ) ) ;
#24268=FACE_OUTER_BOUND ( 'NONE', #24563, .T. ) ;
#24286=CARTESIAN_POINT ( 'NONE',  ( 108.0825317499999869, 107.3738262389971538, -54.72499999726881015 ) ) ;
#24303=EDGE_CURVE ( 'NONE', #7323, #9015, #16213, .T. ) ;
#24319=CARTESIAN_POINT ( 'NONE',  ( 107.0000000000000000, 110.0000000000000000, -145.0000000000000284 ) ) ;
#24320=CARTESIAN_POINT ( 'NONE',  ( 99.99999999999997158, 102.6397644303321215, -55.99999999453763877 ) ) ;
#24335=CARTESIAN_POINT ( 'NONE',  ( 93.46109445667489979, 114.7507929638356785, -50.07499999726882578 ) ) ;
#24364=CARTESIAN_POINT ( 'NONE',  ( 99.99999999999997158, 117.3602355696678501, -49.50000000000002132 ) ) ;
#24390=CARTESIAN_POINT ( 'NONE',  ( 106.5389055433250860, 114.7507929638356785, -46.42499999726882720 ) ) ;
#24392=CARTESIAN_POINT ( 'NONE',  ( 91.91746824999997045, 112.6261737610028320, -51.97499999726882436 ) ) ;
#24414=CARTESIAN_POINT ( 'NONE',  ( 99.99999999999998579, 110.0000000000000000, -145.0000000000000284 ) ) ;
#24424=CIRCLE ( 'NONE', #14391, 5.000000000000004441 ) ;
#24427=CARTESIAN_POINT ( 'NONE',  ( 91.91746824999998466, 110.0000000000000000, -51.62499999726882294 ) ) ;
#24441=AXIS2_PLACEMENT_3D ( 'NONE', #14309, #16461, #3921 ) ;
#24462=AXIS2_PLACEMENT_3D ( 'NONE', #13122, #15269, #8591 ) ;
#24483=CARTESIAN_POINT ( 'NONE',  ( 95.67376207875072680, 104.0454443415356991, -52.70000000000000284 ) ) ;
#24489=CARTESIAN_POINT ( 'NONE',  ( 92.99999999999998579, 112.2744378736303190, -45.10000000000001563 ) ) ;
#24502=EDGE_CURVE ( 'NONE', #22871, #24786, #22785, .T. ) ;
#24510=CARTESIAN_POINT ( 'NONE',  ( 94.33688103937534208, 114.1144967660473242, -53.20000000000000995 ) ) ;
#24515=EDGE_CURVE ( 'NONE', #14596, #8895, #9235, .T. ) ;
#24535=CARTESIAN_POINT ( 'NONE',  ( 106.5389055433250860, 105.2492070361643215, -46.82499999726881867 ) ) ;
#24540=LINE ( 'NONE', #9568, #7936 ) ;
#24563=EDGE_LOOP ( 'NONE', ( #22054, #21560, #5767, #7031 ) ) ;
#24574=CARTESIAN_POINT ( 'NONE',  ( 95.00472066334982912, 103.1245878333314323, -47.57499999726882578 ) ) ;
#24575=ORIENTED_EDGE ( 'NONE', *, *, #19099, .F. ) ;
#24588=( BOUNDED_CURVE ( )  B_SPLINE_CURVE ( 2, ( #11552, #7287, #6866, #13551, #11126, #7003, #26548, #24261, #19990, #9426, #20268 ),
 .UNSPECIFIED., .F., .T. ) 
 B_SPLINE_CURVE_WITH_KNOTS ( ( 3, 2, 2, 2, 2, 3 ),
 ( 0.2000000000000001776, 0.2200000000000001676, 0.2400000000000001854, 0.2600000000000002309, 0.2800000000000002487, 0.3000000000000002109 ),
 .UNSPECIFIED. ) 
 CURVE ( )  GEOMETRIC_REPRESENTATION_ITEM ( )  RATIONAL_B_SPLINE_CURVE ( ( 0.9999999999999995559, 0.9510565162951539753, 1.000000000000000000, 0.9510565162951535312, 1.000000000000000000, 0.9510565162951535312, 1.000000000000000000, 0.9510565162951535312, 1.000000000000000000, 0.9510565162951529761, 1.000000000000000444 ) ) 
 REPRESENTATION_ITEM ( '' )  );
#24624=CARTESIAN_POINT ( 'NONE',  ( 106.5389055433250860, 105.2492070361643215, -51.07499999726882578 ) ) ;
#24658=CARTESIAN_POINT ( 'NONE',  ( 102.1631189606246295, 103.3426043859339103, -54.40000000000001279 ) ) ;
#24690=ORIENTED_EDGE ( 'NONE', *, *, #24303, .T. ) ;
#24718=CARTESIAN_POINT ( 'NONE',  ( 104.9952793366501709, 103.1245878333314323, -51.17499999726881299 ) ) ;
#24763=CARTESIAN_POINT ( 'NONE',  ( 91.91746824999998466, 110.0000000000000000, -55.87499999726882294 ) ) ;
#24786=VERTEX_POINT ( 'NONE', #17367 ) ;
#24792=CARTESIAN_POINT ( 'NONE',  ( 97.83688103937537051, 103.3426043859339103, -54.60000000000000853 ) ) ;
#24800=EDGE_LOOP ( 'NONE', ( #2394, #10446 ) ) ;
#24823=DIRECTION ( 'NONE',  ( 0.000000000000000000, 0.000000000000000000, 1.000000000000000000 ) ) ;
#24842=AXIS2_PLACEMENT_3D ( 'NONE', #25977, #26116, #6448 ) ;
#24848=DIRECTION ( 'NONE',  ( -5.782411586589357392E-17, 0.000000000000000000, -1.000000000000000000 ) ) ;
#24858=CARTESIAN_POINT ( 'NONE',  ( 99.99999999999997158, 118.4984768113314004, -52.37499999726880873 ) ) ;
#24926=CARTESIAN_POINT ( 'NONE',  ( 99.99999999999997158, 118.4984768113314004, -52.37499999726880873 ) ) ;
#24934=CARTESIAN_POINT ( 'NONE',  ( 105.6631189606246153, 114.1144967660473242, -53.80000000000001137 ) ) ;
#24976=AXIS2_PLACEMENT_3D ( 'NONE', #15557, #9292, #17989 ) ;
#24993=EDGE_LOOP ( 'NONE', ( #23672, #8398, #14996, #23351 ) ) ;
#24999=CARTESIAN_POINT ( 'NONE',  ( 97.50236033167490746, 117.6869444889999841, -48.27499999726882152 ) ) ;
#25017=CARTESIAN_POINT ( 'NONE',  ( 97.83688103937535629, 116.6573956140660897, -46.89999999453763735 ) ) ;
#25035=CARTESIAN_POINT ( 'NONE',  ( 107.0000000000000000, 110.0000000000000000, -145.0000000000000284 ) ) ;
#25045=CARTESIAN_POINT ( 'NONE',  ( 102.4976396683250783, 102.3130555110000159, -55.27499999726882152 ) ) ;
#25052=CARTESIAN_POINT ( 'NONE',  ( 95.67376207875072680, 115.9545556584642867, -50.79999999453763593 ) ) ;
#25069=CARTESIAN_POINT ( 'NONE',  ( 91.91746824999997045, 107.3738262389971538, -53.77499999726881441 ) ) ;
#25077=CARTESIAN_POINT ( 'NONE',  ( 105.6631189606246295, 105.8855032339526758, -54.20000000000000995 ) ) ;
#25090=CARTESIAN_POINT ( 'NONE',  ( 91.91746824999998466, 110.0000000000000000, -45.87499999726882294 ) ) ;
#25102=CARTESIAN_POINT ( 'NONE',  ( 102.4976396683250783, 102.3130555110000159, -55.02499999726882152 ) ) ;
#25132=CARTESIAN_POINT ( 'NONE',  ( 93.46109445667489979, 105.2492070361643215, -49.67499999726882010 ) ) ;
#25136=CARTESIAN_POINT ( 'NONE',  ( 93.00000000000000000, 112.2744378736303332, -45.10000000000001563 ) ) ;
#25165=UNCERTAINTY_MEASURE_WITH_UNIT (LENGTH_MEASURE( 1.000000000000000082E-05 ), #10302, 'distance_accuracy_value', 'NONE');
#25179=CARTESIAN_POINT ( 'NONE',  ( 95.00472066334981491, 116.8754121666685393, -52.17499999726882010 ) ) ;
#25186=CARTESIAN_POINT ( 'NONE',  ( 91.91746824999998466, 110.0000000000000000, -55.74999999726882294 ) ) ;
#25205=CARTESIAN_POINT ( 'NONE',  ( 104.3262379212492448, 104.0454443415356991, -47.79999999453763593 ) ) ;
#25208=CARTESIAN_POINT ( 'NONE',  ( 95.67376207875072680, 104.0454443415356991, -52.19999999453764161 ) ) ;
#25213=CARTESIAN_POINT ( 'NONE',  ( 99.99999999999997158, 118.4984768113314004, -52.12499999726880873 ) ) ;
#25215=ORIENTED_EDGE ( 'NONE', *, *, #6469, .T. ) ;
#25236=CARTESIAN_POINT ( 'NONE',  ( 91.91746824999997045, 107.3738262389971680, -55.52499999726881441 ) ) ;
#25269=CARTESIAN_POINT ( 'NONE',  ( 107.0000000000000000, 110.0000000000000000, -49.49999999453764588 ) ) ;
#25270=CARTESIAN_POINT ( 'NONE',  ( 91.91746824999998466, 110.0000000000000000, -55.87499999726882294 ) ) ;
#25279=EDGE_LOOP ( 'NONE', ( #14134, #26075, #106, #21111, #17939, #3552, #14152, #22414, #9251, #18995, #25707, #19713, #24575 ) ) ;
#25288=CARTESIAN_POINT ( 'NONE',  ( 105.6631189606246153, 114.1144967660473242, -47.29999999453764303 ) ) ;
#25303=CARTESIAN_POINT ( 'NONE',  ( 102.4976396683250783, 102.3130555110000159, -49.02499999726882152 ) ) ;
#25334=DIRECTION ( 'NONE',  ( -1.000000000000000000, 0.000000000000000000, 0.000000000000000000 ) ) ;
#25340=VECTOR ( 'NONE', #7805, 1000.000000000000000 ) ;
#25344=CARTESIAN_POINT ( 'NONE',  ( 94.33688103937534208, 114.1144967660473242, -50.69999999453764161 ) ) ;
#25356=CARTESIAN_POINT ( 'NONE',  ( 104.9952793366501709, 116.8754121666685393, -50.32499999726882578 ) ) ;
#25364=CIRCLE ( 'NONE', #3963, 5.000000000000004441 ) ;
#25365=CARTESIAN_POINT ( 'NONE',  ( 92.99999999999998579, 110.0000000000000000, -145.0000000000000284 ) ) ;
#25368=CARTESIAN_POINT ( 'NONE',  ( 92.99999999999998579, 110.0000000000000000, -50.49999999453763877 ) ) ;
#25415=FILL_AREA_STYLE_COLOUR ( '', #15887 ) ;
#25447=CARTESIAN_POINT ( 'NONE',  ( 93.46109445667489979, 105.2492070361643215, -49.42499999726882010 ) ) ;
#25484=CARTESIAN_POINT ( 'NONE',  ( 104.3262379212492448, 115.9545556584642867, -51.19999999453763451 ) ) ;
#25492=CARTESIAN_POINT ( 'NONE',  ( 102.4976396683250783, 102.3130555110000159, -53.02499999726882862 ) ) ;
#25611=DIRECTION ( 'NONE',  ( 1.000000000000000000, 0.000000000000000000, 0.000000000000000000 ) ) ;
#25616=CARTESIAN_POINT ( 'NONE',  ( 99.99999999999997158, 102.6397644303321215, -53.99999999453763877 ) ) ;
#25625=CARTESIAN_POINT ( 'NONE',  ( 97.50236033167490746, 117.6869444889999841, -54.02499999726882862 ) ) ;
#25636=CARTESIAN_POINT ( 'NONE',  ( 107.0000000000000000, 110.0000000000000000, -48.00000000000001421 ) ) ;
#25649=ORIENTED_EDGE ( 'NONE', *, *, #22584, .T. ) ;
#25662=( BOUNDED_CURVE ( )  B_SPLINE_CURVE ( 2, ( #14044, #11190, #7493, #9634, #18340, #11477, #20194, #679, #4809, #393, #20485 ),
 .UNSPECIFIED., .F., .F. ) 
 B_SPLINE_CURVE_WITH_KNOTS ( ( 3, 2, 2, 2, 2, 3 ),
 ( 0.5999999999999998668, 0.6199999999999998845, 0.6399999999999999023, 0.6599999999999999201, 0.6799999999999999378, 0.6999999999999998446 ),
 .UNSPECIFIED. ) 
 CURVE ( )  GEOMETRIC_REPRESENTATION_ITEM ( )  RATIONAL_B_SPLINE_CURVE ( ( 1.000000000000000222, 0.9510565162951533091, 1.000000000000000000, 0.9510565162951535312, 1.000000000000000000, 0.9510565162951535312, 1.000000000000000000, 0.9510565162951535312, 1.000000000000000000, 0.9510565162951537532, 0.9999999999999997780 ) ) 
 REPRESENTATION_ITEM ( '' )  );
#25672=CARTESIAN_POINT ( 'NONE',  ( 92.99999999999998579, 110.0000000000000000, -55.74999999726883004 ) ) ;
#25679=CARTESIAN_POINT ( 'NONE',  ( 91.91746824999998466, 110.0000000000000000, -45.62499999726882294 ) ) ;
#25687=CARTESIAN_POINT ( 'NONE',  ( 99.99999999999997158, 101.5015231886685854, -55.37499999726883004 ) ) ;
#25707=ORIENTED_EDGE ( 'NONE', *, *, #16663, .T. ) ;
#25717=CARTESIAN_POINT ( 'NONE',  ( 93.46109445667489979, 105.2492070361643215, -47.42499999726882720 ) ) ;
#25755=CARTESIAN_POINT ( 'NONE',  ( 102.1631189606246295, 103.3426043859339103, -51.89999999453764445 ) ) ;
#25763=CARTESIAN_POINT ( 'NONE',  ( 106.5389055433250860, 105.2492070361643215, -50.82499999726882578 ) ) ;
#25775=( BOUNDED_SURFACE ( )  B_SPLINE_SURFACE ( 1, 2, ( 
 ( #27295, #25136, #28084, #8547, #14292, #20592, #21250, #14803, #16302, #1075, #23526, #1732, #10396, #4004, #12670, #21395, #1873, #10537, #6970, #17380, #17810, #13222, #2433, #431, #6828, #26513, #15082, #13367, #11235, #2147, #4852, #19953, #12937, #26369, #9115, #17663, #17950, #24226, #17521, #19524, #21670, #10809, #4560, #5, #4280, #24364, #22096, #15226, #22238, #15518, #15665, #2717, #11378, #13517, #20099, #26078, #15369, #576, #8690, #24086, #21954, #6546, #9257, #6413, #23944, #2574, #23802, #4424, #13078, #21817, #6683, #2293, #10952, #19663, #4707, #146, #8831, #26224, #11093, #19805, #289, #8974, #24510, #20670, #13661, #13940, #14228, #1154, #24934, #16377, #3277, #9540, #25077, #20529, #24658, #2848, #24792, #18090, #7392, #4998, #18241 ),
 ( #26660, #718, #11946, #20805, #11806, #5565, #5274, #22521, #3412, #14090, #7252, #11517, #22376, #9819, #1285, #22666, #5421, #3138, #26949, #15942, #16086, #27231, #18526, #5131, #1011, #7685, #22950, #9680, #12081, #18383, #9953, #27088, #13797, #7539, #16237, #7107, #22809, #2986, #15805, #11660, #20236, #9393, #26802, #20382, #868, #10505, #1974, #25356, #1702, #19211, #27368, #23494, #25763, #27504, #16793, #10221, #12492, #7960, #21493, #7827, #23635, #6245, #14914, #12361, #27639, #25213, #16659, #8375, #18666, #20944, #3974, #12777, #3830, #17060, #25492, #14506, #4111, #6107, #5837, #23084, #5701, #12634, #16520, #5972, #25625, #23357, #18931, #23223, #8100, #27914, #21361, #3699, #1568, #1842, #14368, #14639, #3558, #21218, #12216, #10360, #21079 ) ),
 .UNSPECIFIED., .F., .F., .T. ) 
 B_SPLINE_SURFACE_WITH_KNOTS ( ( 2, 2 ),
 ( 3, 2, 2, 2, 2, 2, 2, 2, 2, 2, 2, 2, 2, 2, 2, 2, 2, 2, 2, 2, 2, 2, 2, 2, 2, 2, 2, 2, 2, 2, 2, 2, 2, 2, 2, 2, 2, 2, 2, 2, 2, 2, 2, 2, 2, 2, 2, 2, 2, 2, 3 ),
 ( 0.000000000000000000, 1.000000000000000000 ),
 ( 0.000000000000000000, 0.02000000000000000042, 0.04000000000000000083, 0.05999999999999999778, 0.08000000000000000167, 0.1000000000000000056, 0.1199999999999999956, 0.1400000000000000133, 0.1600000000000000033, 0.1799999999999999933, 0.2000000000000000111, 0.2200000000000000011, 0.2399999999999999911, 0.2600000000000000089, 0.2800000000000000266, 0.2999999999999999889, 0.3200000000000000067, 0.3400000000000000244, 0.3599999999999999867, 0.3800000000000000044, 0.4000000000000000222, 0.4199999999999999845, 0.4400000000000000022, 0.4600000000000000200, 0.4799999999999999822, 0.5000000000000000000, 0.5200000000000000178, 0.5400000000000000355, 0.5600000000000000533, 0.5799999999999999600, 0.5999999999999999778, 0.6199999999999999956, 0.6400000000000000133, 0.6600000000000000311, 0.6800000000000000488, 0.6999999999999999556, 0.7199999999999999734, 0.7399999999999999911, 0.7600000000000000089, 0.7800000000000000266, 0.8000000000000000444, 0.8199999999999999512, 0.8399999999999999689, 0.8599999999999999867, 0.8800000000000000044, 0.9000000000000000222, 0.9200000000000000400, 0.9399999999999999467, 0.9599999999999999645, 0.9799999999999999822, 1.000000000000000000 ),
 .UNSPECIFIED. ) 
 GEOMETRIC_REPRESENTATION_ITEM ( )  RATIONAL_B_SPLINE_SURFACE ( (
 ( 1.000000000000000000, 0.9510565162951535312, 1.000000000000000000, 0.9510565162951535312, 1.000000000000000000, 0.9510565162951535312, 1.000000000000000000, 0.9510565162951535312, 1.000000000000000000, 0.9510565162951535312, 1.000000000000000000, 0.9510565162951535312, 1.000000000000000000, 0.9510565162951535312, 1.000000000000000000, 0.9510565162951535312, 1.000000000000000000, 0.9510565162951535312, 1.000000000000000000, 0.9510565162951535312, 1.000000000000000000, 0.9510565162951535312, 1.000000000000000000, 0.9510565162951535312, 1.000000000000000000, 0.9510565162951535312, 1.000000000000000000, 0.9510565162951535312, 1.000000000000000000, 0.9510565162951535312, 1.000000000000000000, 0.9510565162951535312, 1.000000000000000000, 0.9510565162951535312, 1.000000000000000000, 0.9510565162951535312, 1.000000000000000000, 0.9510565162951535312, 1.000000000000000000, 0.9510565162951535312, 1.000000000000000000, 0.9510565162951535312, 1.000000000000000000, 0.9510565162951535312, 1.000000000000000000, 0.9510565162951535312, 1.000000000000000000, 0.9510565162951535312, 1.000000000000000000, 0.9510565162951535312, 1.000000000000000000, 0.9510565162951535312, 1.000000000000000000, 0.9510565162951535312, 1.000000000000000000, 0.9510565162951535312, 1.000000000000000000, 0.9510565162951535312, 1.000000000000000000, 0.9510565162951535312, 1.000000000000000000, 0.9510565162951535312, 1.000000000000000000, 0.9510565162951535312, 1.000000000000000000, 0.9510565162951535312, 1.000000000000000000, 0.9510565162951535312, 1.000000000000000000, 0.9510565162951535312, 1.000000000000000000, 0.9510565162951535312, 1.000000000000000000, 0.9510565162951535312, 1.000000000000000000, 0.9510565162951535312, 1.000000000000000000, 0.9510565162951535312, 1.000000000000000000, 0.9510565162951535312, 1.000000000000000000, 0.9510565162951535312, 1.000000000000000000, 0.9510565162951535312, 1.000000000000000000, 0.9510565162951535312, 1.000000000000000000, 0.9510565162951535312, 1.000000000000000000, 0.9510565162951535312, 1.000000000000000000, 0.9510565162951535312, 1.000000000000000000, 0.9510565162951535312, 1.000000000000000000, 0.9510565162951535312, 1.000000000000000000, 0.9510565162951535312, 1.000000000000000000, 0.9510565162951535312, 1.000000000000000000),
 ( 1.000000000000000000, 0.9510565162951535312, 1.000000000000000000, 0.9510565162951535312, 1.000000000000000000, 0.9510565162951535312, 1.000000000000000000, 0.9510565162951535312, 1.000000000000000000, 0.9510565162951535312, 1.000000000000000000, 0.9510565162951535312, 1.000000000000000000, 0.9510565162951535312, 1.000000000000000000, 0.9510565162951535312, 1.000000000000000000, 0.9510565162951535312, 1.000000000000000000, 0.9510565162951535312, 1.000000000000000000, 0.9510565162951535312, 1.000000000000000000, 0.9510565162951535312, 1.000000000000000000, 0.9510565162951535312, 1.000000000000000000, 0.9510565162951535312, 1.000000000000000000, 0.9510565162951535312, 1.000000000000000000, 0.9510565162951535312, 1.000000000000000000, 0.9510565162951535312, 1.000000000000000000, 0.9510565162951535312, 1.000000000000000000, 0.9510565162951535312, 1.000000000000000000, 0.9510565162951535312, 1.000000000000000000, 0.9510565162951535312, 1.000000000000000000, 0.9510565162951535312, 1.000000000000000000, 0.9510565162951535312, 1.000000000000000000, 0.9510565162951535312, 1.000000000000000000, 0.9510565162951535312, 1.000000000000000000, 0.9510565162951535312, 1.000000000000000000, 0.9510565162951535312, 1.000000000000000000, 0.9510565162951535312, 1.000000000000000000, 0.9510565162951535312, 1.000000000000000000, 0.9510565162951535312, 1.000000000000000000, 0.9510565162951535312, 1.000000000000000000, 0.9510565162951535312, 1.000000000000000000, 0.9510565162951535312, 1.000000000000000000, 0.9510565162951535312, 1.000000000000000000, 0.9510565162951535312, 1.000000000000000000, 0.9510565162951535312, 1.000000000000000000, 0.9510565162951535312, 1.000000000000000000, 0.9510565162951535312, 1.000000000000000000, 0.9510565162951535312, 1.000000000000000000, 0.9510565162951535312, 1.000000000000000000, 0.9510565162951535312, 1.000000000000000000, 0.9510565162951535312, 1.000000000000000000, 0.9510565162951535312, 1.000000000000000000, 0.9510565162951535312, 1.000000000000000000, 0.9510565162951535312, 1.000000000000000000, 0.9510565162951535312, 1.000000000000000000, 0.9510565162951535312, 1.000000000000000000, 0.9510565162951535312, 1.000000000000000000, 0.9510565162951535312, 1.000000000000000000, 0.9510565162951535312, 1.000000000000000000) ) ) 
 REPRESENTATION_ITEM ( '' )  SURFACE ( )  );
#25810=ADVANCED_FACE ( 'NONE', ( #19407 ), #8381, .F. ) ;
#25824=CARTESIAN_POINT ( 'NONE',  ( 95.00472066334982912, 116.8754121666685393, -48.17499999726882010 ) ) ;
#25835=CARTESIAN_POINT ( 'NONE',  ( 107.0000000000000000, 110.0000000000000000, -54.00000000000001421 ) ) ;
#25847=EDGE_CURVE ( 'NONE', #17997, #20267, #10369, .T. ) ;
#25851=SHAPE_REPRESENTATION_RELATIONSHIP ( 'NONE' , 'NONE' ,  #14947, #4607 ) ;
#25861=CARTESIAN_POINT ( 'NONE',  ( 102.4976396683250783, 117.6869444889999841, -48.22499999726881725 ) ) ;
#25863=EDGE_CURVE ( 'NONE', #21015, #12194, #3657, .T. ) ;
#25881=PLANE ( 'NONE',  #14270 ) ;
#25901=CARTESIAN_POINT ( 'NONE',  ( 99.99999999999997158, 117.3602355696678501, -50.99999999453762456 ) ) ;
#25904=CARTESIAN_POINT ( 'NONE',  ( 97.83688103937537051, 103.3426043859339103, -56.09999999453764730 ) ) ;
#25967=CARTESIAN_POINT ( 'NONE',  ( 102.4976396683250783, 102.3130555110000159, -51.27499999726882152 ) ) ;
#25977=CARTESIAN_POINT ( 'NONE',  ( 99.99999999999998579, 110.0000000000000000, -145.0000000000000284 ) ) ;
#26001=CARTESIAN_POINT ( 'NONE',  ( 106.5389055433250860, 114.7507929638356785, -52.42499999726882010 ) ) ;
#26036=CARTESIAN_POINT ( 'NONE',  ( 93.00000000000000000, 107.7255621263696526, -56.39999999453763024 ) ) ;
#26049=CARTESIAN_POINT ( 'NONE',  ( 99.99999999999997158, 118.4984768113314146, -48.37499999726881583 ) ) ;
#26052=VECTOR ( 'NONE', #5396, 1000.000000000000000 ) ;
#26056=CARTESIAN_POINT ( 'NONE',  ( 107.0000000000000000, 110.0000000000000000, -47.49999999453763877 ) ) ;
#26075=ORIENTED_EDGE ( 'NONE', *, *, #6201, .T. ) ;
#26077=( BOUNDED_CURVE ( )  B_SPLINE_CURVE ( 2, ( #25835, #12976, #4179, #27984, #19560, #16992, #6040, #17133, #12841, #2043, #6309 ),
 .UNSPECIFIED., .F., .F. ) 
 B_SPLINE_CURVE_WITH_KNOTS ( ( 3, 2, 2, 2, 2, 3 ),
 ( 0.9000000000000000222, 0.9200000000000000400, 0.9399999999999999467, 0.9599999999999999645, 0.9799999999999999822, 1.000000000000000000 ),
 .UNSPECIFIED. ) 
 CURVE ( )  GEOMETRIC_REPRESENTATION_ITEM ( )  RATIONAL_B_SPLINE_CURVE ( ( 1.000000000000000000, 0.9510565162951535312, 1.000000000000000000, 0.9510565162951535312, 1.000000000000000000, 0.9510565162951535312, 1.000000000000000000, 0.9510565162951535312, 1.000000000000000000, 0.9510565162951535312, 1.000000000000000000 ) ) 
 REPRESENTATION_ITEM ( '' )  );
#26078=CARTESIAN_POINT ( 'NONE',  ( 99.99999999999997158, 102.6397644303321215, -50.50000000000000000 ) ) ;
#26100=CARTESIAN_POINT ( 'NONE',  ( 99.99999999999998579, 110.0000000000000000, -145.0000000000000284 ) ) ;
#26105=CARTESIAN_POINT ( 'NONE',  ( 91.91746824999997045, 112.6261737610028320, -49.72499999726882436 ) ) ;
#26107=CARTESIAN_POINT ( 'NONE',  ( 93.46109445667489979, 105.2492070361643215, -49.67499999726882010 ) ) ;
#26116=DIRECTION ( 'NONE',  ( 5.782411586589358625E-17, -0.000000000000000000, 1.000000000000000000 ) ) ;
#26129=ORIENTED_EDGE ( 'NONE', *, *, #24303, .F. ) ;
#26141=CARTESIAN_POINT ( 'NONE',  ( 97.50236033167490746, 117.6869444889999841, -52.02499999726882862 ) ) ;
#26157=FACE_OUTER_BOUND ( 'NONE', #24800, .T. ) ;
#26176=CARTESIAN_POINT ( 'NONE',  ( 107.0000000000000000, 112.2744378736303190, -55.39999999453763735 ) ) ;
#26188=CARTESIAN_POINT ( 'NONE',  ( 104.9952793366501567, 116.8754121666685393, -46.57499999726881157 ) ) ;
#26224=CARTESIAN_POINT ( 'NONE',  ( 95.67376207875069838, 104.0454443415356991, -52.70000000000000284 ) ) ;
#26238=EDGE_LOOP ( 'NONE', ( #21035, #25649, #15729, #19408 ) ) ;
#26250=CARTESIAN_POINT ( 'NONE',  ( 102.4976396683250783, 117.6869444889999841, -46.22499999726882436 ) ) ;
#26253=CARTESIAN_POINT ( 'NONE',  ( 108.0825317499999869, 107.3738262389971538, -50.97499999726881015 ) ) ;
#26282=PRODUCT ( 'main air inlet', 'main air inlet', '', ( #27929 ) ) ;
#26289=CARTESIAN_POINT ( 'NONE',  ( 97.50236033167490746, 102.3130555110000159, -53.22499999726882436 ) ) ;
#26325=CARTESIAN_POINT ( 'NONE',  ( 102.1631189606246153, 116.6573956140660897, -55.09999999453764019 ) ) ;
#26369=CARTESIAN_POINT ( 'NONE',  ( 104.3262379212492448, 104.0454443415356991, -48.30000000000001137 ) ) ;
#26386=COLOUR_RGB ( '', 0.66274510, 0.83137255, 0.94901961) ;
#26397=CARTESIAN_POINT ( 'NONE',  ( 91.91746824999997045, 107.3738262389971680, -49.52499999726881441 ) ) ;
#26399=CARTESIAN_POINT ( 'NONE',  ( 95.00472066334982912, 103.1245878333314323, -53.57499999726881157 ) ) ;
#26434=CARTESIAN_POINT ( 'NONE',  ( 108.0825317499999869, 112.6261737610028320, -54.52499999726880731 ) ) ;
#26484=CARTESIAN_POINT ( 'NONE',  ( 95.00472066334981491, 103.1245878333314465, -47.57499999726882578 ) ) ;
#26513=CARTESIAN_POINT ( 'NONE',  ( 99.99999999999997158, 117.3602355696678501, -47.50000000000001421 ) ) ;
#26537=CARTESIAN_POINT ( 'NONE',  ( 99.99999999999997158, 101.5015231886685712, -47.12499999726882294 ) ) ;
#26540=CARTESIAN_POINT ( 'NONE',  ( 91.91746824999997045, 107.3738262389971538, -55.77499999726882862 ) ) ;
#26548=CARTESIAN_POINT ( 'NONE',  ( 102.1631189606246153, 116.6573956140660897, -49.09999999453764019 ) ) ;
#26577=CARTESIAN_POINT ( 'NONE',  ( 91.91746824999998466, 110.0000000000000000, -55.62499999726882294 ) ) ;
#26605=ADVANCED_FACE ( 'NONE', ( #3067 ), #11732, .T. ) ;
#26629=CARTESIAN_POINT ( 'NONE',  ( 97.50236033167490746, 102.3130555110000159, -47.47499999726881725 ) ) ;
#26660=CARTESIAN_POINT ( 'NONE',  ( 91.91746824999998466, 110.0000000000000000, -45.62499999726882294 ) ) ;
#26663=EDGE_LOOP ( 'NONE', ( #22200, #376, #5200, #13430 ) ) ;
#26685=CARTESIAN_POINT ( 'NONE',  ( 95.00472066334981491, 116.8754121666685393, -51.92499999726881299 ) ) ;
#26721=CARTESIAN_POINT ( 'NONE',  ( 108.0825317499999869, 112.6261737610028320, -50.77499999726882152 ) ) ;
#26772=CARTESIAN_POINT ( 'NONE',  ( 104.9952793366501567, 116.8754121666685393, -50.57499999726882578 ) ) ;
#26797=FACE_OUTER_BOUND ( 'NONE', #19034, .T. ) ;
#26802=CARTESIAN_POINT ( 'NONE',  ( 93.46109445667489979, 114.7507929638356785, -49.82499999726882578 ) ) ;
#26824=CARTESIAN_POINT ( 'NONE',  ( 92.45873412499997812, 110.0000000000000000, -56.18749999590323796 ) ) ;
#26832=CARTESIAN_POINT ( 'NONE',  ( 93.46109445667489979, 105.2492070361643215, -53.42499999726882720 ) ) ;
#26844=AXIS2_PLACEMENT_3D ( 'NONE', #8635, #24028, #23608 ) ;
#26869=CARTESIAN_POINT ( 'NONE',  ( 91.91746824999997045, 107.3738262389971538, -51.77499999726881441 ) ) ;
#26898=CARTESIAN_POINT ( 'NONE',  ( 104.3262379212492448, 115.9545556584642867, -53.19999999453762740 ) ) ;
#26915=CARTESIAN_POINT ( 'NONE',  ( 106.5389055433250860, 114.7507929638356785, -54.67499999726882720 ) ) ;
#26920=CARTESIAN_POINT ( 'NONE',  ( 92.99999999999998579, 110.0000000000000000, -53.00000000000001421 ) ) ;
#26944=CARTESIAN_POINT ( 'NONE',  ( 104.3262379212492448, 115.9545556584642867, -47.70000000000000995 ) ) ;
#26949=CARTESIAN_POINT ( 'NONE',  ( 93.46109445667489979, 105.2492070361643215, -47.42499999726882720 ) ) ;
#27009=CARTESIAN_POINT ( 'NONE',  ( 93.46109445667489979, 114.7507929638356785, -52.07499999726881867 ) ) ;
#27056=CARTESIAN_POINT ( 'NONE',  ( 97.50236033167490746, 102.3130555110000159, -55.47499999726881725 ) ) ;
#27078=CARTESIAN_POINT ( 'NONE',  ( 99.99999999999997158, 101.5015231886685854, -53.37499999726883004 ) ) ;
#27082=CARTESIAN_POINT ( 'NONE',  ( 92.99999999999998579, 110.0000000000000000, -47.00000000000001421 ) ) ;
#27088=CARTESIAN_POINT ( 'NONE',  ( 108.0825317499999869, 107.3738262389971538, -48.72499999726881015 ) ) ;
#27115=CARTESIAN_POINT ( 'NONE',  ( 102.4976396683250783, 117.6869444889999841, -54.22499999726881725 ) ) ;
#27154=DIRECTION ( 'NONE',  ( 5.782411586589358625E-17, -0.000000000000000000, 1.000000000000000000 ) ) ;
#27155=CARTESIAN_POINT ( 'NONE',  ( 99.99999999999997158, 101.5015231886685854, -47.37499999726882294 ) ) ;
#27185=CARTESIAN_POINT ( 'NONE',  ( 107.0000000000000000, 110.0000000000000000, -50.00000000000000711 ) ) ;
#27202=CARTESIAN_POINT ( 'NONE',  ( 108.0825317500000011, 110.0000000000000000, -54.87499999726882294 ) ) ;
#27219=CARTESIAN_POINT ( 'NONE',  ( 92.99999999999998579, 107.7255621263696952, -46.90000000000002700 ) ) ;
#27220=VERTEX_POINT ( 'NONE', #25090 ) ;
#27222=CARTESIAN_POINT ( 'NONE',  ( 97.50236033167490746, 102.3130555110000159, -55.47499999726881725 ) ) ;
#27224=EDGE_LOOP ( 'NONE', ( #22901, #2974, #1289, #3026 ) ) ;
#27225=CARTESIAN_POINT ( 'NONE',  ( 92.99999999999998579, 110.0000000000000000, -52.49999999453763877 ) ) ;
#27231=CARTESIAN_POINT ( 'NONE',  ( 91.91746824999997045, 112.6261737610028320, -47.72499999726881725 ) ) ;
#27236=VERTEX_POINT ( 'NONE', #25368 ) ;
#27247=LINE ( 'NONE', #26824, #23666 ) ;
#27254=CARTESIAN_POINT ( 'NONE',  ( 108.0825317499999869, 107.3738262389971680, -54.72499999726881015 ) ) ;
#27291=CARTESIAN_POINT ( 'NONE',  ( 102.4976396683250783, 102.3130555110000159, -49.27499999726882152 ) ) ;
#27295=CARTESIAN_POINT ( 'NONE',  ( 92.99999999999998579, 110.0000000000000000, -45.00000000000001421 ) ) ;
#27336=CARTESIAN_POINT ( 'NONE',  ( 104.9952793366501567, 103.1245878333314465, -51.17499999726881299 ) ) ;
#27361=CARTESIAN_POINT ( 'NONE',  ( 104.9952793366501709, 103.1245878333314323, -55.17499999726882720 ) ) ;
#27368=CARTESIAN_POINT ( 'NONE',  ( 108.0825317500000011, 110.0000000000000000, -50.62499999726882294 ) ) ;
#27409=CARTESIAN_POINT ( 'NONE',  ( 107.0000000000000142, 107.7255621263696952, -50.10000000000000853 ) ) ;
#27417=SURFACE_STYLE_USAGE ( .BOTH. , #5897 ) ;
#27421=CARTESIAN_POINT ( 'NONE',  ( 108.0825317499999869, 107.3738262389971538, -54.97499999726881015 ) ) ;
#27453=CARTESIAN_POINT ( 'NONE',  ( 106.5389055433250860, 105.2492070361643215, -48.82499999726882578 ) ) ;
#27495=CYLINDRICAL_SURFACE ( 'NONE', #7683, 7.000000000000006217 ) ;
#27496=CARTESIAN_POINT ( 'NONE',  ( 94.33688103937535629, 105.8855032339526758, -54.29999999453764303 ) ) ;
#27504=CARTESIAN_POINT ( 'NONE',  ( 104.9952793366501709, 103.1245878333314323, -50.92499999726882010 ) ) ;
#27511=LINE ( 'NONE', #25365, #3806 ) ;
#27534=ORIENTED_EDGE ( 'NONE', *, *, #2626, .T. ) ;
#27542=CARTESIAN_POINT ( 'NONE',  ( 102.1631189606246153, 116.6573956140660897, -53.60000000000000853 ) ) ;
#27591=CARTESIAN_POINT ( 'NONE',  ( 106.5389055433250860, 105.2492070361643215, -46.82499999726881867 ) ) ;
#27600=LINE ( 'NONE', #3795, #7959 ) ;
#27619=EDGE_LOOP ( 'NONE', ( #6677, #10507, #20285, #8317, #22622, #583, #19780, #22587, #15700, #2201, #8405, #26129, #9716 ) ) ;
#27630=CARTESIAN_POINT ( 'NONE',  ( 97.83688103937535629, 116.6573956140660897, -52.89999999453764445 ) ) ;
#27634=CARTESIAN_POINT ( 'NONE',  ( 107.0000000000000000, 110.0000000000000000, -51.49999999453763877 ) ) ;
#27639=CARTESIAN_POINT ( 'NONE',  ( 97.50236033167490746, 117.6869444889999841, -52.02499999726882862 ) ) ;
#27653=CARTESIAN_POINT ( 'NONE',  ( 95.67376207875072680, 104.0454443415356991, -48.70000000000000995 ) ) ;
#27768=CARTESIAN_POINT ( 'NONE',  ( 97.83688103937535629, 116.6573956140660897, -48.89999999453763735 ) ) ;
#27771=CARTESIAN_POINT ( 'NONE',  ( 104.3262379212492448, 104.0454443415356991, -51.79999999453762882 ) ) ;
#27790=CARTESIAN_POINT ( 'NONE',  ( 105.6631189606246295, 105.8855032339526758, -48.20000000000001705 ) ) ;
#27817=ORIENTED_EDGE ( 'NONE', *, *, #6927, .F. ) ;
#27838=CARTESIAN_POINT ( 'NONE',  ( 106.5389055433250860, 114.7507929638356785, -46.67499999726882720 ) ) ;
#27843=CARTESIAN_POINT ( 'NONE',  ( 102.4976396683250783, 117.6869444889999841, -54.47499999726881725 ) ) ;
#27905=CARTESIAN_POINT ( 'NONE',  ( 102.1631189606246153, 116.6573956140660897, -51.09999999453764019 ) ) ;
#27914=CARTESIAN_POINT ( 'NONE',  ( 108.0825317499999869, 112.6261737610028320, -54.52499999726880731 ) ) ;
#27929=PRODUCT_CONTEXT ( 'NONE', #21529, 'mechanical' ) ;
#27973=CARTESIAN_POINT ( 'NONE',  ( 97.50236033167490746, 102.3130555110000159, -49.47499999726882436 ) ) ;
#27976=CARTESIAN_POINT ( 'NONE',  ( 92.99999999999998579, 107.7255621263696526, -54.39999999453763024 ) ) ;
#27978=CARTESIAN_POINT ( 'NONE',  ( 108.0825317500000011, 110.0000000000000000, -52.87499999726882294 ) ) ;
#27984=CARTESIAN_POINT ( 'NONE',  ( 104.3262379212492448, 104.0454443415356991, -54.30000000000001137 ) ) ;
#28008=CARTESIAN_POINT ( 'NONE',  ( 108.0825317500000011, 110.0000000000000000, -46.62499999726882294 ) ) ;
#28044=CARTESIAN_POINT ( 'NONE',  ( 105.6631189606246153, 114.1144967660473242, -51.29999999453763593 ) ) ;
#28047=CARTESIAN_POINT ( 'NONE',  ( 107.0000000000000000, 110.0000000000000000, -55.49999999453763877 ) ) ;
#28084=CARTESIAN_POINT ( 'NONE',  ( 94.33688103937534208, 114.1144967660473242, -45.20000000000000995 ) ) ;
#28104=DIRECTION ( 'NONE',  ( 5.782411586589358625E-17, -0.000000000000000000, 1.000000000000000000 ) ) ;
#28130=DIRECTION ( 'NONE',  ( 5.782411586589358625E-17, -0.000000000000000000, 1.000000000000000000 ) ) ;
#28144=CARTESIAN_POINT ( 'NONE',  ( 108.0825317500000011, 110.0000000000000000, -52.62499999726882294 ) ) ;
#28180=CARTESIAN_POINT ( 'NONE',  ( 105.6631189606246295, 105.8855032339526758, -55.69999999453764161 ) ) ;
#28184=CARTESIAN_POINT ( 'NONE',  ( 102.1631189606246295, 103.3426043859339103, -55.89999999453763735 ) ) ;
#28196=DIRECTION ( 'NONE',  ( 1.000000000000000000, 0.000000000000000000, 0.000000000000000000 ) ) ;
ENDSEC;
END-ISO-10303-21;
